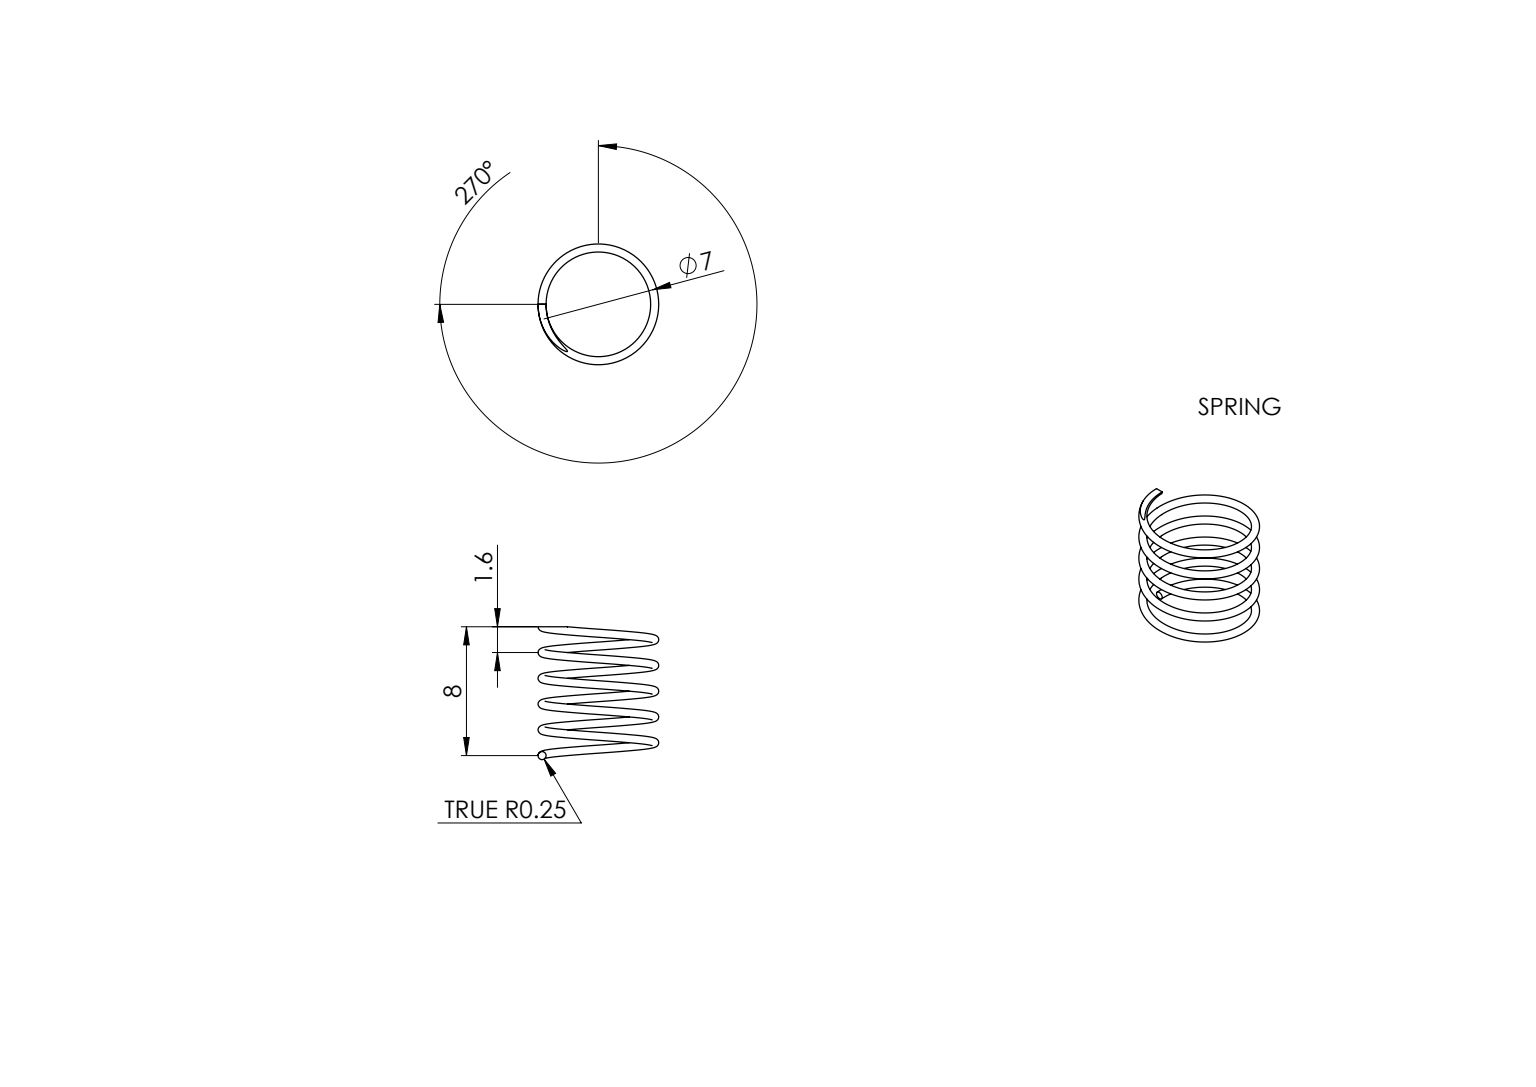
ISO-10303-21;
HEADER;
FILE_DESCRIPTION (('STEP AP214'),
    '1' );
FILE_NAME ('spring.step',
    '2026-10-27T10:49:47',
    ( '' ),
    ( '' ),
    'SwSTEP 2.0',
    'SolidWorks 2026',
    '' );
FILE_SCHEMA (( 'AUTOMOTIVE_DESIGN' ));
ENDSEC;

DATA;
#5=CARTESIAN_POINT ( 'NONE',  ( -2.108492589042352261, -1.550659073900639395, 2.134148098076933397 ) ) ;
#11=( NAMED_UNIT ( * ) SI_UNIT ( $, .STERADIAN. ) SOLID_ANGLE_UNIT ( ) );
#15=CARTESIAN_POINT ( 'NONE',  ( -2.593667801677444817, -2.017599804162952387E-16, 2.576081167903025104 ) ) ;
#18=CARTESIAN_POINT ( 'NONE',  ( -1.467888652719046449, -6.949340926099361049, 3.492485675378536047 ) ) ;
#25=CARTESIAN_POINT ( 'NONE',  ( 0.01814118441313990887, -6.550659073900639839, 3.500000000000000000 ) ) ;
#33=CARTESIAN_POINT ( 'NONE',  ( 3.492485675378536047, -0.9493409260993610488, 1.467888652719046672 ) ) ;
#36=CARTESIAN_POINT ( 'NONE',  ( 1.260781871532495657, -2.949340926099361937, -2.992485675378538268 ) ) ;
#40=CARTESIAN_POINT ( 'NONE',  ( 1.638713065079247855, -2.450659073900638862, -4.007514324621431534 ) ) ;
#50=CARTESIAN_POINT ( 'NONE',  ( 2.992485675378565357, -0.6506590739006395951, -1.260781871532430376 ) ) ;
#59=CARTESIAN_POINT ( 'NONE',  ( -2.110065146580993645, -1.191525181865938352E-11, 2.889420178070662093 ) ) ;
#61=CARTESIAN_POINT ( 'NONE',  ( -1.431606283892620235, -7.949340926099361049, -3.507514324621463953 ) ) ;
#62=CARTESIAN_POINT ( 'NONE',  ( -1.467888652719046449, -3.749340926099360871, 3.492485675378536047 ) ) ;
#69=CARTESIAN_POINT ( 'NONE',  ( 2.487701488670203354, -6.750659073900639129, 2.462045979635629323 ) ) ;
#77=CARTESIAN_POINT ( 'NONE',  ( -3.507514324621464397, -0.3493409260993610710, 1.431606283892619347 ) ) ;
#78=CARTESIAN_POINT ( 'NONE',  ( -3.000000000000000444, -5.049340926099361582, -0.01814118441320822922 ) ) ;
#82=CARTESIAN_POINT ( 'NONE',  ( 0.01814118441321938349, -1.449340926099360827, -4.000000000000000000 ) ) ;
#90=CARTESIAN_POINT ( 'NONE',  ( 2.134148098076933397, -5.150659073900639484, 2.108492589042352261 ) ) ;
#104=CARTESIAN_POINT ( 'NONE',  ( 3.492485675378536047, -7.349340926099362292, 1.467888652719046672 ) ) ;
#114=CARTESIAN_POINT ( 'NONE',  ( -4.000000000000000000, -7.750659073900639129, 0.01814118441313491634 ) ) ;
#122=CARTESIAN_POINT ( 'NONE',  ( -2.487701488670255312, -2.049340926099361582, 2.462045979635577808 ) ) ;
#125=CARTESIAN_POINT ( 'NONE',  ( 3.000000000000000444, -5.849340926099360516, 0.01814118441320859698 ) ) ;
#127=CARTESIAN_POINT ( 'NONE',  ( -1.674995433905599462, -0.5493409260993608045, 3.992485675378533383 ) ) ;
#138=CARTESIAN_POINT ( 'NONE',  ( 3.007514324621436863, -6.850659073900641438, 1.224499502706140719 ) ) ;
#139=ORIENTED_EDGE ( 'NONE', *, *, #8501, .F. ) ;
#149=CARTESIAN_POINT ( 'NONE',  ( 1.431606283892619125, -5.549340926099361582, 3.507514324621464397 ) ) ;
#152=CARTESIAN_POINT ( 'NONE',  ( -1.467888652719046449, -6.949340926099361049, 3.492485675378536047 ) ) ;
#155=CARTESIAN_POINT ( 'NONE',  ( 2.487701488670203354, -6.750659073900639129, 2.462045979635629323 ) ) ;
#156=AXIS2_PLACEMENT_3D ( 'NONE', #2203, #2343, #5173 ) ;
#161=CARTESIAN_POINT ( 'NONE',  ( -1.674995433905516196, -5.850659073900638774, -3.992485675378566690 ) ) ;
#169=CARTESIAN_POINT ( 'NONE',  ( 2.462045979635577364, -2.449340926099361049, 2.487701488670255312 ) ) ;
#171=CARTESIAN_POINT ( 'NONE',  ( 1.224499502706142273, -2.450659073900639751, -3.007514324621435531 ) ) ;
#174=CARTESIAN_POINT ( 'NONE',  ( -2.815599370228846876, -1.649340926099360560, -2.841254879263533262 ) ) ;
#177=CARTESIAN_POINT ( 'NONE',  ( 2.462045979635577364, -0.8493409260993610710, 2.487701488670255312 ) ) ;
#181=CARTESIAN_POINT ( 'NONE',  ( -1.674995433905599462, -5.349340926099361404, 3.992485675378533383 ) ) ;
#183=VERTEX_POINT ( 'NONE', #6311 ) ;
#185=CARTESIAN_POINT ( 'NONE',  ( 2.992485675378565357, -5.450659073900638418, -1.260781871532430376 ) ) ;
#195=CARTESIAN_POINT ( 'NONE',  ( 1.467888652719048226, -1.349340926099361182, -3.492485675378536047 ) ) ;
#203=CARTESIAN_POINT ( 'NONE',  ( 3.507514324621434199, -6.850659073900639662, 1.431606283892693066 ) ) ;
#211=CARTESIAN_POINT ( 'NONE',  ( -3.992485675378568022, -3.050659073900638951, 1.674995433905515529 ) ) ;
#219=CARTESIAN_POINT ( 'NONE',  ( -3.000000000000000444, 0.2493409260993606213, 0.01814118441314532468 ) ) ;
#223=CARTESIAN_POINT ( 'NONE',  ( 1.674995433905601239, -1.349340926099360960, -3.992485675378532939 ) ) ;
#224=( BOUNDED_SURFACE ( )  B_SPLINE_SURFACE ( 3, 2, ( 
 ( #862, #77, #7899, #2314, #3760, #7195, #3662, #33, #7151, #5702, #1518, #3711, #8682, #6487, #6589, #4994, #6536, #6398, #122, #8546, #2971, #5140, #169, #8636, #2266, #7944, #7851, #1565, #2618, #4787, #7676, #3958, #2660, #1914, #3403, #6785, #1117, #8281, #411, #1259, #1961, #1297, #6886, #559, #1872, #4052, #7630, #1212, #2704, #4098, #3259, #6231, #4005, #5387, #4739, #8237, #4140, #6931, #8418, #6085, #9063, #514, #3357, #3307, #3445, #7586, #5533, #6973, #6187, #6138, #8968, #5435, #5573, #8377, #463, #9015, #5482, #2004, #2569, #8330, #8920 ),
 ( #4830, #602, #6272, #4650, #9107, #2752, #7491, #4695, #1161, #7533, #6839, #4365, #5615, #2973, #6489, #3664, #5046, #6401, #684, #1520, #8590, #7198, #3576, #7811, #8508, #728, #7153, #36, #6809, #2176, #7901, #1345, #2887, #2133, #776, #4184, #7718, #5662, #7016, #7853, #8548, #822, #4269, #3622, #8463, #1428, #4996, #7105, #78, #1474, #642, #6445, #1385, #2796, #4956, #2091, #125, #4317, #5798, #3488, #2929, #5703, #5749, #3531, #2045, #2220, #4870, #6313, #9149, #6355, #2842, #4915, #7763, #4230, #7061, #6591, #5191, #5981, #6538, #4451, #7946 ),
 ( #219, #3207, #5284, #5143, #7290, #3762, #8823, #7381, #8131, #2459, #1568, #915, #8637, #3071, #6680, #1007, #355, #8084, #8778, #4505, #5890, #3856, #3021, #7433, #3902, #5845, #1059, #171, #864, #3808, #4549, #6723, #4409, #8684, #309, #2408, #3161, #1711, #7336, #2268, #2316, #8730, #5096, #7239, #4595, #2362, #8033, #1664, #962, #7985, #6634, #262, #3713, #1613, #1759, #3115, #5938, #5238, #3250, #4128, #3995, #6073, #6962, #4779, #402, #7666, #3299, #593, #4088, #3948, #6026, #2695, #2557, #4686, #1152, #3392, #7621, #5522, #6221, #5327, #1861 ),
 ( #1248, #8863, #5472, #6177, #1903, #7523, #6923, #8910, #4822, #1288, #5377, #2503, #6775, #7478, #1202, #1949, #8180, #1809, #8228, #549, #9004, #9051, #8319, #4731, #4640, #6828, #6126, #1108, #453, #1994, #8957, #2608, #5424, #8272, #7573, #4044, #6876, #504, #3347, #8368, #2650, #7093, #4259, #633, #1510, #1376, #3477, #4354, #2166, #7008, #5034, #675, #7189, #1460, #1332, #8539, #1419, #4219, #3565, #6434, #2744, #717, #3519, #4986, #5564, #9096, #7051, #8409, #25, #6389, #69, #5650, #7843, #6304, #2831, #2873, #9179, #4307, #5694, #2036, #7143 ),
 ( #4174, #766, #6345, #9141, #2785, #4859, #2920, #5737, #8498, #4903, #7891, #3608, #8582, #2210, #3436, #5605, #8450, #2077, #7754, #2120, #4946, #7707, #6265, #7802, #995, #5083, #6479, #6578, #8767, #952, #7371, #299, #2350, #211, #7279, #8718, #6624, #4494, #3153, #251, #5180, #1601, #4584, #5971, #3061, #8022, #2307, #5227, #906, #5881, #1654, #8675, #5785, #3102, #5129, #5835, #3842, #6668, #7325, #3801, #7937, #161, #1558, #7976, #5927, #8071, #3753, #8812, #7228, #2398, #811, #4442, #5275, #1701, #4538, #2449, #3011, #8119, #1748, #3654, #114 ),
 ( #2963, #8627, #2258, #4398, #855, #3702, #6527, #343, #1045, #3893, #6713, #3196, #7421, #4559, #1017, #7998, #366, #6735, #2514, #230, #1069, #8740, #877, #7444, #8143, #1625, #3171, #7346, #5154, #6601, #3727, #3911, #3215, #8045, #2374, #8873, #2468, #7394, #6688, #8094, #3079, #5901, #925, #3774, #3818, #5203, #6551, #6035, #1673, #5340, #2326, #181, #6643, #5993, #3865, #1722, #4516, #8189, #1818, #7251, #3035, #5292, #972, #272, #318, #5855, #4464, #8695, #7302, #3125, #5949, #2419, #8788, #5249, #8832, #1770, #4605, #1982, #8994, #8441, #625 ),
 ( #1940, #4813, #4769, #667, #3467, #4937, #6868, #6296, #6256, #3427, #9042, #9172, #1280, #5597, #3512, #7658, #2684, #5514, #4119, #2112, #7697, #6213, #8357, #6953, #7745, #8309, #583, #492, #9088, #7613, #3339, #2729, #1190, #7043, #6915, #5556, #8400, #1369, #9132, #6335, #4209, #6168, #2028, #4034, #4851, #2066, #2776, #2642, #4894, #1322, #4165, #6999, #2820, #1237, #5640, #8490, #4079, #5463, #539, #3380, #2954, #3690, #3052, #707, #4978, #6515, #1548, #152, #7218, #3645, #7795, #2158, #7879, #5869, #8709, #3745, #5727, #61, #5022, #2910, #8530 ) ),
 .UNSPECIFIED., .T., .F., .T. ) 
 B_SPLINE_SURFACE_WITH_KNOTS ( ( 4, 3, 4 ),
 ( 3, 2, 2, 2, 2, 2, 2, 2, 2, 2, 2, 2, 2, 2, 2, 2, 2, 2, 2, 2, 2, 2, 2, 2, 2, 2, 2, 2, 2, 2, 2, 2, 2, 2, 2, 2, 2, 2, 2, 2, 3 ),
 ( 0.000000000000000000, 0.5000000000000000000, 1.000000000000000000 ),
 ( 0.000000000000000000, 0.02500000000000000139, 0.05000000000000000278, 0.07499999999999999722, 0.1000000000000000056, 0.1250000000000000000, 0.1499999999999999944, 0.1749999999999999889, 0.2000000000000000111, 0.2250000000000000056, 0.2500000000000000000, 0.2750000000000000222, 0.2999999999999999889, 0.3250000000000000111, 0.3499999999999999778, 0.3750000000000000000, 0.4000000000000000222, 0.4249999999999999889, 0.4500000000000000111, 0.4749999999999999778, 0.5000000000000000000, 0.5250000000000000222, 0.5500000000000000444, 0.5749999999999999556, 0.5999999999999999778, 0.6250000000000000000, 0.6500000000000000222, 0.6750000000000000444, 0.6999999999999999556, 0.7249999999999999778, 0.7500000000000000000, 0.7750000000000000222, 0.8000000000000000444, 0.8249999999999999556, 0.8499999999999999778, 0.8750000000000000000, 0.9000000000000000222, 0.9250000000000000444, 0.9499999999999999556, 0.9749999999999999778, 1.000000000000000000 ),
 .UNSPECIFIED. ) 
 GEOMETRIC_REPRESENTATION_ITEM ( )  RATIONAL_B_SPLINE_SURFACE ( (
 ( 1.000000000000000000, 0.9238795325112867385, 1.000000000000000000, 0.9238795325112867385, 1.000000000000000000, 0.9238795325112867385, 1.000000000000000000, 0.9238795325112867385, 1.000000000000000000, 0.9238795325112867385, 1.000000000000000000, 0.9238795325112867385, 1.000000000000000000, 0.9238795325112867385, 1.000000000000000000, 0.9238795325112867385, 1.000000000000000000, 0.9238795325112867385, 1.000000000000000000, 0.9238795325112867385, 1.000000000000000000, 0.9238795325112867385, 1.000000000000000000, 0.9238795325112867385, 1.000000000000000000, 0.9238795325112867385, 1.000000000000000000, 0.9238795325112867385, 1.000000000000000000, 0.9238795325112867385, 1.000000000000000000, 0.9238795325112867385, 1.000000000000000000, 0.9238795325112867385, 1.000000000000000000, 0.9238795325112867385, 1.000000000000000000, 0.9238795325112867385, 1.000000000000000000, 0.9238795325112867385, 1.000000000000000000, 0.9238795325112867385, 1.000000000000000000, 0.9238795325112867385, 1.000000000000000000, 0.9238795325112867385, 1.000000000000000000, 0.9238795325112867385, 1.000000000000000000, 0.9238795325112867385, 1.000000000000000000, 0.9238795325112867385, 1.000000000000000000, 0.9238795325112867385, 1.000000000000000000, 0.9238795325112867385, 1.000000000000000000, 0.9238795325112867385, 1.000000000000000000, 0.9238795325112867385, 1.000000000000000000, 0.9238795325112867385, 1.000000000000000000, 0.9238795325112867385, 1.000000000000000000, 0.9238795325112867385, 1.000000000000000000, 0.9238795325112867385, 1.000000000000000000, 0.9238795325112867385, 1.000000000000000000, 0.9238795325112867385, 1.000000000000000000, 0.9238795325112867385, 1.000000000000000000, 0.9238795325112867385, 1.000000000000000000, 0.9238795325112867385, 1.000000000000000000, 0.9238795325112867385, 1.000000000000000000),
 ( 0.3333333333333333703, 0.3079598441704289313, 0.3333333333333333703, 0.3079598441704289313, 0.3333333333333333703, 0.3079598441704289313, 0.3333333333333333703, 0.3079598441704289313, 0.3333333333333333703, 0.3079598441704289313, 0.3333333333333333703, 0.3079598441704289313, 0.3333333333333333703, 0.3079598441704289313, 0.3333333333333333703, 0.3079598441704289313, 0.3333333333333333703, 0.3079598441704289313, 0.3333333333333333703, 0.3079598441704289313, 0.3333333333333333703, 0.3079598441704289313, 0.3333333333333333703, 0.3079598441704289313, 0.3333333333333333703, 0.3079598441704289313, 0.3333333333333333703, 0.3079598441704289313, 0.3333333333333333703, 0.3079598441704289313, 0.3333333333333333703, 0.3079598441704289313, 0.3333333333333333703, 0.3079598441704289313, 0.3333333333333333703, 0.3079598441704289313, 0.3333333333333333703, 0.3079598441704289313, 0.3333333333333333703, 0.3079598441704289313, 0.3333333333333333703, 0.3079598441704289313, 0.3333333333333333703, 0.3079598441704289313, 0.3333333333333333703, 0.3079598441704289313, 0.3333333333333333703, 0.3079598441704289313, 0.3333333333333333703, 0.3079598441704289313, 0.3333333333333333703, 0.3079598441704289313, 0.3333333333333333703, 0.3079598441704289313, 0.3333333333333333703, 0.3079598441704289313, 0.3333333333333333703, 0.3079598441704289313, 0.3333333333333333703, 0.3079598441704289313, 0.3333333333333333703, 0.3079598441704289313, 0.3333333333333333703, 0.3079598441704289313, 0.3333333333333333703, 0.3079598441704289313, 0.3333333333333333703, 0.3079598441704289313, 0.3333333333333333703, 0.3079598441704289313, 0.3333333333333333703, 0.3079598441704289313, 0.3333333333333333703, 0.3079598441704289313, 0.3333333333333333703, 0.3079598441704289313, 0.3333333333333333703, 0.3079598441704289313, 0.3333333333333333703, 0.3079598441704289313, 0.3333333333333333703),
 ( 0.3333333333333333703, 0.3079598441704289313, 0.3333333333333333703, 0.3079598441704289313, 0.3333333333333333703, 0.3079598441704289313, 0.3333333333333333703, 0.3079598441704289313, 0.3333333333333333703, 0.3079598441704289313, 0.3333333333333333703, 0.3079598441704289313, 0.3333333333333333703, 0.3079598441704289313, 0.3333333333333333703, 0.3079598441704289313, 0.3333333333333333703, 0.3079598441704289313, 0.3333333333333333703, 0.3079598441704289313, 0.3333333333333333703, 0.3079598441704289313, 0.3333333333333333703, 0.3079598441704289313, 0.3333333333333333703, 0.3079598441704289313, 0.3333333333333333703, 0.3079598441704289313, 0.3333333333333333703, 0.3079598441704289313, 0.3333333333333333703, 0.3079598441704289313, 0.3333333333333333703, 0.3079598441704289313, 0.3333333333333333703, 0.3079598441704289313, 0.3333333333333333703, 0.3079598441704289313, 0.3333333333333333703, 0.3079598441704289313, 0.3333333333333333703, 0.3079598441704289313, 0.3333333333333333703, 0.3079598441704289313, 0.3333333333333333703, 0.3079598441704289313, 0.3333333333333333703, 0.3079598441704289313, 0.3333333333333333703, 0.3079598441704289313, 0.3333333333333333703, 0.3079598441704289313, 0.3333333333333333703, 0.3079598441704289313, 0.3333333333333333703, 0.3079598441704289313, 0.3333333333333333703, 0.3079598441704289313, 0.3333333333333333703, 0.3079598441704289313, 0.3333333333333333703, 0.3079598441704289313, 0.3333333333333333703, 0.3079598441704289313, 0.3333333333333333703, 0.3079598441704289313, 0.3333333333333333703, 0.3079598441704289313, 0.3333333333333333703, 0.3079598441704289313, 0.3333333333333333703, 0.3079598441704289313, 0.3333333333333333703, 0.3079598441704289313, 0.3333333333333333703, 0.3079598441704289313, 0.3333333333333333703, 0.3079598441704289313, 0.3333333333333333703, 0.3079598441704289313, 0.3333333333333333703),
 ( 1.000000000000000000, 0.9238795325112867385, 1.000000000000000000, 0.9238795325112867385, 1.000000000000000000, 0.9238795325112867385, 1.000000000000000000, 0.9238795325112867385, 1.000000000000000000, 0.9238795325112867385, 1.000000000000000000, 0.9238795325112867385, 1.000000000000000000, 0.9238795325112867385, 1.000000000000000000, 0.9238795325112867385, 1.000000000000000000, 0.9238795325112867385, 1.000000000000000000, 0.9238795325112867385, 1.000000000000000000, 0.9238795325112867385, 1.000000000000000000, 0.9238795325112867385, 1.000000000000000000, 0.9238795325112867385, 1.000000000000000000, 0.9238795325112867385, 1.000000000000000000, 0.9238795325112867385, 1.000000000000000000, 0.9238795325112867385, 1.000000000000000000, 0.9238795325112867385, 1.000000000000000000, 0.9238795325112867385, 1.000000000000000000, 0.9238795325112867385, 1.000000000000000000, 0.9238795325112867385, 1.000000000000000000, 0.9238795325112867385, 1.000000000000000000, 0.9238795325112867385, 1.000000000000000000, 0.9238795325112867385, 1.000000000000000000, 0.9238795325112867385, 1.000000000000000000, 0.9238795325112867385, 1.000000000000000000, 0.9238795325112867385, 1.000000000000000000, 0.9238795325112867385, 1.000000000000000000, 0.9238795325112867385, 1.000000000000000000, 0.9238795325112867385, 1.000000000000000000, 0.9238795325112867385, 1.000000000000000000, 0.9238795325112867385, 1.000000000000000000, 0.9238795325112867385, 1.000000000000000000, 0.9238795325112867385, 1.000000000000000000, 0.9238795325112867385, 1.000000000000000000, 0.9238795325112867385, 1.000000000000000000, 0.9238795325112867385, 1.000000000000000000, 0.9238795325112867385, 1.000000000000000000, 0.9238795325112867385, 1.000000000000000000, 0.9238795325112867385, 1.000000000000000000, 0.9238795325112867385, 1.000000000000000000),
 ( 0.3333333333333333703, 0.3079598441704289313, 0.3333333333333333703, 0.3079598441704289313, 0.3333333333333333703, 0.3079598441704289313, 0.3333333333333333703, 0.3079598441704289313, 0.3333333333333333703, 0.3079598441704289313, 0.3333333333333333703, 0.3079598441704289313, 0.3333333333333333703, 0.3079598441704289313, 0.3333333333333333703, 0.3079598441704289313, 0.3333333333333333703, 0.3079598441704289313, 0.3333333333333333703, 0.3079598441704289313, 0.3333333333333333703, 0.3079598441704289313, 0.3333333333333333703, 0.3079598441704289313, 0.3333333333333333703, 0.3079598441704289313, 0.3333333333333333703, 0.3079598441704289313, 0.3333333333333333703, 0.3079598441704289313, 0.3333333333333333703, 0.3079598441704289313, 0.3333333333333333703, 0.3079598441704289313, 0.3333333333333333703, 0.3079598441704289313, 0.3333333333333333703, 0.3079598441704289313, 0.3333333333333333703, 0.3079598441704289313, 0.3333333333333333703, 0.3079598441704289313, 0.3333333333333333703, 0.3079598441704289313, 0.3333333333333333703, 0.3079598441704289313, 0.3333333333333333703, 0.3079598441704289313, 0.3333333333333333703, 0.3079598441704289313, 0.3333333333333333703, 0.3079598441704289313, 0.3333333333333333703, 0.3079598441704289313, 0.3333333333333333703, 0.3079598441704289313, 0.3333333333333333703, 0.3079598441704289313, 0.3333333333333333703, 0.3079598441704289313, 0.3333333333333333703, 0.3079598441704289313, 0.3333333333333333703, 0.3079598441704289313, 0.3333333333333333703, 0.3079598441704289313, 0.3333333333333333703, 0.3079598441704289313, 0.3333333333333333703, 0.3079598441704289313, 0.3333333333333333703, 0.3079598441704289313, 0.3333333333333333703, 0.3079598441704289313, 0.3333333333333333703, 0.3079598441704289313, 0.3333333333333333703, 0.3079598441704289313, 0.3333333333333333703, 0.3079598441704289313, 0.3333333333333333703),
 ( 0.3333333333333333703, 0.3079598441704289313, 0.3333333333333333703, 0.3079598441704289313, 0.3333333333333333703, 0.3079598441704289313, 0.3333333333333333703, 0.3079598441704289313, 0.3333333333333333703, 0.3079598441704289313, 0.3333333333333333703, 0.3079598441704289313, 0.3333333333333333703, 0.3079598441704289313, 0.3333333333333333703, 0.3079598441704289313, 0.3333333333333333703, 0.3079598441704289313, 0.3333333333333333703, 0.3079598441704289313, 0.3333333333333333703, 0.3079598441704289313, 0.3333333333333333703, 0.3079598441704289313, 0.3333333333333333703, 0.3079598441704289313, 0.3333333333333333703, 0.3079598441704289313, 0.3333333333333333703, 0.3079598441704289313, 0.3333333333333333703, 0.3079598441704289313, 0.3333333333333333703, 0.3079598441704289313, 0.3333333333333333703, 0.3079598441704289313, 0.3333333333333333703, 0.3079598441704289313, 0.3333333333333333703, 0.3079598441704289313, 0.3333333333333333703, 0.3079598441704289313, 0.3333333333333333703, 0.3079598441704289313, 0.3333333333333333703, 0.3079598441704289313, 0.3333333333333333703, 0.3079598441704289313, 0.3333333333333333703, 0.3079598441704289313, 0.3333333333333333703, 0.3079598441704289313, 0.3333333333333333703, 0.3079598441704289313, 0.3333333333333333703, 0.3079598441704289313, 0.3333333333333333703, 0.3079598441704289313, 0.3333333333333333703, 0.3079598441704289313, 0.3333333333333333703, 0.3079598441704289313, 0.3333333333333333703, 0.3079598441704289313, 0.3333333333333333703, 0.3079598441704289313, 0.3333333333333333703, 0.3079598441704289313, 0.3333333333333333703, 0.3079598441704289313, 0.3333333333333333703, 0.3079598441704289313, 0.3333333333333333703, 0.3079598441704289313, 0.3333333333333333703, 0.3079598441704289313, 0.3333333333333333703, 0.3079598441704289313, 0.3333333333333333703, 0.3079598441704289313, 0.3333333333333333703),
 ( 1.000000000000000000, 0.9238795325112867385, 1.000000000000000000, 0.9238795325112867385, 1.000000000000000000, 0.9238795325112867385, 1.000000000000000000, 0.9238795325112867385, 1.000000000000000000, 0.9238795325112867385, 1.000000000000000000, 0.9238795325112867385, 1.000000000000000000, 0.9238795325112867385, 1.000000000000000000, 0.9238795325112867385, 1.000000000000000000, 0.9238795325112867385, 1.000000000000000000, 0.9238795325112867385, 1.000000000000000000, 0.9238795325112867385, 1.000000000000000000, 0.9238795325112867385, 1.000000000000000000, 0.9238795325112867385, 1.000000000000000000, 0.9238795325112867385, 1.000000000000000000, 0.9238795325112867385, 1.000000000000000000, 0.9238795325112867385, 1.000000000000000000, 0.9238795325112867385, 1.000000000000000000, 0.9238795325112867385, 1.000000000000000000, 0.9238795325112867385, 1.000000000000000000, 0.9238795325112867385, 1.000000000000000000, 0.9238795325112867385, 1.000000000000000000, 0.9238795325112867385, 1.000000000000000000, 0.9238795325112867385, 1.000000000000000000, 0.9238795325112867385, 1.000000000000000000, 0.9238795325112867385, 1.000000000000000000, 0.9238795325112867385, 1.000000000000000000, 0.9238795325112867385, 1.000000000000000000, 0.9238795325112867385, 1.000000000000000000, 0.9238795325112867385, 1.000000000000000000, 0.9238795325112867385, 1.000000000000000000, 0.9238795325112867385, 1.000000000000000000, 0.9238795325112867385, 1.000000000000000000, 0.9238795325112867385, 1.000000000000000000, 0.9238795325112867385, 1.000000000000000000, 0.9238795325112867385, 1.000000000000000000, 0.9238795325112867385, 1.000000000000000000, 0.9238795325112867385, 1.000000000000000000, 0.9238795325112867385, 1.000000000000000000, 0.9238795325112867385, 1.000000000000000000, 0.9238795325112867385, 1.000000000000000000) ) ) 
 REPRESENTATION_ITEM ( '' )  SURFACE ( )  );
#227=CARTESIAN_POINT ( 'NONE',  ( -0.01814118441321365544, -0.6493409260993610044, 3.500000000000000000 ) ) ;
#230=CARTESIAN_POINT ( 'NONE',  ( -1.674995433905599462, -2.149340926099360782, 3.992485675378533383 ) ) ;
#234=CARTESIAN_POINT ( 'NONE',  ( -1.260781871532431708, -5.850659073900641438, -2.992485675378564469 ) ) ;
#240=CARTESIAN_POINT ( 'NONE',  ( -1.467888652719046449, -3.749340926099360871, 3.492485675378536047 ) ) ;
#251=CARTESIAN_POINT ( 'NONE',  ( 4.007514324621432422, -3.650659073900639040, 1.638713065079246078 ) ) ;
#254=ORIENTED_EDGE ( 'NONE', *, *, #8365, .F. ) ;
#262=CARTESIAN_POINT ( 'NONE',  ( -1.224499502706140497, -4.850659073900639662, 3.007514324621436863 ) ) ;
#266=DIRECTION ( 'NONE',  ( 0.000000000000000000, -0.9973637043974449279, -0.07256473765270717025 ) ) ;
#267=CARTESIAN_POINT ( 'NONE',  ( 0.01814118441321408565, -1.449340926099361271, -3.500000000000000000 ) ) ;
#272=CARTESIAN_POINT ( 'NONE',  ( -3.992485675378532939, -6.549340926099361582, -1.674995433905601683 ) ) ;
#276=CARTESIAN_POINT ( 'NONE',  ( 0.01814118441314514080, -4.950659073900641083, 3.000000000000000444 ) ) ;
#280=CARTESIAN_POINT ( 'NONE',  ( -1.041183273768722772, -0.07758948893217661180, 3.505490685814065088 ) ) ;
#285=CARTESIAN_POINT ( 'NONE',  ( -2.487701488670255312, -2.049340926099361582, 2.462045979635577808 ) ) ;
#295=AXIS2_PLACEMENT_3D ( 'NONE', #3494, #5755, #4370 ) ;
#299=CARTESIAN_POINT ( 'NONE',  ( -4.007514324621431534, -2.850659073900638774, -1.638713065079248521 ) ) ;
#309=CARTESIAN_POINT ( 'NONE',  ( -2.108492589042352261, -3.150659073900639484, 2.134148098076933397 ) ) ;
#318=CARTESIAN_POINT ( 'NONE',  ( -4.000000000000000000, -6.649340926099362115, -0.01814118441321865144 ) ) ;
#322=CARTESIAN_POINT ( 'NONE',  ( 0.01814118441313990887, -6.550659073900639839, 3.500000000000000000 ) ) ;
#329=EDGE_LOOP ( 'NONE', ( #5209, #4297, #1353, #1594, #6573 ) ) ;
#332=CARTESIAN_POINT ( 'NONE',  ( -0.01814118441321365544, -5.449340926099361937, 3.500000000000000000 ) ) ;
#341=DIRECTION ( 'NONE',  ( 0.000000000000000000, -0.000000000000000000, 1.000000000000000000 ) ) ;
#343=CARTESIAN_POINT ( 'NONE',  ( 3.992485675378533383, -0.9493409260993608267, 1.674995433905599462 ) ) ;
#355=CARTESIAN_POINT ( 'NONE',  ( -3.000000000000000444, -1.350659073900639440, 0.01814118441314532468 ) ) ;
#361=CARTESIAN_POINT ( 'NONE',  ( -3.500000000000000000, -0.2493409260993610654, -0.01814118441321343686 ) ) ;
#364=PRODUCT_CONTEXT ( 'NONE', #1831, 'mechanical' ) ;
#366=CARTESIAN_POINT ( 'NONE',  ( -4.000000000000000000, -1.849340926099360738, -0.01814118441321865144 ) ) ;
#371=CARTESIAN_POINT ( 'NONE',  ( 1.431606283892694842, -5.650659073900638596, -3.507514324621434199 ) ) ;
#380=CARTESIAN_POINT ( 'NONE',  ( 0.01814118441321408565, -7.849340926099360516, -3.500000000000000000 ) ) ;
#395=CARTESIAN_POINT ( 'NONE',  ( -2.841254879263533262, -0.4493409260993607157, 2.815599370228847764 ) ) ;
#402=CARTESIAN_POINT ( 'NONE',  ( -3.000000000000000444, -6.150659073900639484, 0.01814118441314532468 ) ) ;
#411=CARTESIAN_POINT ( 'NONE',  ( 2.462045979635577364, -4.049340926099360694, 2.487701488670255312 ) ) ;
#414=CARTESIAN_POINT ( 'NONE',  ( 3.492485675378566690, -7.050659073900641616, -1.467888652718972287 ) ) ;
#420=CARTESIAN_POINT ( 'NONE',  ( 3.492485675378566690, -0.6506590739006392621, -1.467888652718972287 ) ) ;
#426=CARTESIAN_POINT ( 'NONE',  ( -1.260781871532494103, -0.5493409260993613596, 2.992485675378538712 ) ) ;
#444=CARTESIAN_POINT ( 'NONE',  ( -1.638713065079163034, -6.349340926099361404, -4.007514324621466173 ) ) ;
#453=CARTESIAN_POINT ( 'NONE',  ( -0.01814118441313947866, -2.550659073900638951, -3.500000000000000000 ) ) ;
#463=CARTESIAN_POINT ( 'NONE',  ( 2.487701488670255756, -7.649340926099361226, -2.462045979635577364 ) ) ;
#466=CARTESIAN_POINT ( 'NONE',  ( 2.462045979635629767, -3.950659073900639751, -2.487701488670203354 ) ) ;
#470=CARTESIAN_POINT ( 'NONE',  ( 2.487701488670203354, -3.550659073900638951, 2.462045979635629323 ) ) ;
#477=CARTESIAN_POINT ( 'NONE',  ( -0.01814118441321365544, -7.049340926099361582, 3.500000000000000000 ) ) ;
#492=CARTESIAN_POINT ( 'NONE',  ( 1.467888652719048226, -2.949340926099361493, -3.492485675378536047 ) ) ;
#493=CARTESIAN_POINT ( 'NONE',  ( -2.815599370228846876, -6.449340926099361049, -2.841254879263533262 ) ) ;
#496=ADVANCED_FACE ( 'NONE', ( #7809 ), #224, .T. ) ;
#504=CARTESIAN_POINT ( 'NONE',  ( 1.467888652718972731, -3.450659073900638862, 3.492485675378566246 ) ) ;
#509=CARTESIAN_POINT ( 'NONE',  ( -3.507514324621464397, -6.749340926099361759, 1.431606283892619569 ) ) ;
#514=CARTESIAN_POINT ( 'NONE',  ( -1.431606283892620235, -6.349340926099360516, -3.507514324621463953 ) ) ;
#518=CARTESIAN_POINT ( 'NONE',  ( 2.487701488670203354, -3.550659073900638951, 2.462045979635629323 ) ) ;
#522=CARTESIAN_POINT ( 'NONE',  ( 3.500000000000000000, -5.350659073900638774, -0.01814118441313969030 ) ) ;
#527=CARTESIAN_POINT ( 'NONE',  ( 2.462045979635577364, -7.249340926099360871, 2.487701488670255312 ) ) ;
#531=( BOUNDED_CURVE ( )  B_SPLINE_CURVE ( 2, ( #361, #7438, #3211, #2413, #227, #6638, #177, #5198, #7991, #1813, #7388, #1621, #267, #6730, #5244, #8784, #8088, #2368, #5288, #7341, #5942, #966, #4644, #871, #4458, #3860, #6682, #4600, #1715, #3075, #4512, #8690, #3029, #7296, #6029, #920, #4554, #3166, #3770, #3720, #8040, #5896, #6545, #3120, #1765, #8828, #8736, #3813, #5987, #2463, #8137, #8868, #6597, #1063, #3907, #5851, #2507, #1669, #5569, #2748, #554, #3953, #4092, #4782, #1293, #509, #3397, #1999, #2700, #8276, #6078, #3352, #4134, #1113, #6182, #6131, #5528, #6225, #8414, #6928, #7624 ),
 .UNSPECIFIED., .F., .T. ) 
 B_SPLINE_CURVE_WITH_KNOTS ( ( 3, 2, 2, 2, 2, 2, 2, 2, 2, 2, 2, 2, 2, 2, 2, 2, 2, 2, 2, 2, 2, 2, 2, 2, 2, 2, 2, 2, 2, 2, 2, 2, 2, 2, 2, 2, 2, 2, 2, 2, 3 ),
 ( 0.000000000000000000, 0.02500000000000000139, 0.05000000000000000278, 0.07499999999999999722, 0.1000000000000000056, 0.1250000000000000000, 0.1499999999999999944, 0.1749999999999999889, 0.2000000000000000111, 0.2250000000000000056, 0.2500000000000000000, 0.2750000000000000222, 0.2999999999999999889, 0.3250000000000000111, 0.3499999999999999778, 0.3750000000000000000, 0.4000000000000000222, 0.4249999999999999889, 0.4500000000000000111, 0.4749999999999999778, 0.5000000000000000000, 0.5250000000000000222, 0.5500000000000000444, 0.5749999999999999556, 0.5999999999999999778, 0.6250000000000000000, 0.6500000000000000222, 0.6750000000000000444, 0.6999999999999999556, 0.7249999999999999778, 0.7500000000000000000, 0.7750000000000000222, 0.8000000000000000444, 0.8249999999999999556, 0.8499999999999999778, 0.8750000000000000000, 0.9000000000000000222, 0.9250000000000000444, 0.9499999999999999556, 0.9749999999999999778, 1.000000000000000000 ),
 .UNSPECIFIED. ) 
 CURVE ( )  GEOMETRIC_REPRESENTATION_ITEM ( )  RATIONAL_B_SPLINE_CURVE ( ( 1.000000000000000000, 0.9238795325112867385, 1.000000000000000000, 0.9238795325112867385, 1.000000000000000000, 0.9238795325112867385, 1.000000000000000000, 0.9238795325112867385, 1.000000000000000000, 0.9238795325112867385, 1.000000000000000000, 0.9238795325112867385, 1.000000000000000000, 0.9238795325112867385, 1.000000000000000000, 0.9238795325112867385, 1.000000000000000000, 0.9238795325112867385, 1.000000000000000000, 0.9238795325112867385, 1.000000000000000000, 0.9238795325112867385, 1.000000000000000000, 0.9238795325112867385, 1.000000000000000000, 0.9238795325112867385, 1.000000000000000000, 0.9238795325112867385, 1.000000000000000000, 0.9238795325112867385, 1.000000000000000000, 0.9238795325112867385, 1.000000000000000000, 0.9238795325112867385, 1.000000000000000000, 0.9238795325112867385, 1.000000000000000000, 0.9238795325112867385, 1.000000000000000000, 0.9238795325112867385, 1.000000000000000000, 0.9238795325112867385, 1.000000000000000000, 0.9238795325112867385, 1.000000000000000000, 0.9238795325112867385, 1.000000000000000000, 0.9238795325112867385, 1.000000000000000000, 0.9238795325112867385, 1.000000000000000000, 0.9238795325112867385, 1.000000000000000000, 0.9238795325112867385, 1.000000000000000000, 0.9238795325112867385, 1.000000000000000000, 0.9238795325112867385, 1.000000000000000000, 0.9238795325112867385, 1.000000000000000000, 0.9238795325112867385, 1.000000000000000000, 0.9238795325112867385, 1.000000000000000000, 0.9238795325112867385, 1.000000000000000000, 0.9238795325112867385, 1.000000000000000000, 0.9238795325112867385, 1.000000000000000000, 0.9238795325112867385, 1.000000000000000000, 0.9238795325112867385, 1.000000000000000000, 0.9238795325112867385, 1.000000000000000000, 0.9238795325112867385, 1.000000000000000000, 0.9238795325112867385, 1.000000000000000000 ) ) 
 REPRESENTATION_ITEM ( '' )  );
#539=CARTESIAN_POINT ( 'NONE',  ( 2.487701488670255756, -6.049340926099361582, -2.462045979635577364 ) ) ;
#540=CARTESIAN_POINT ( 'NONE',  ( 3.992485675378533383, -5.749340926099361759, 1.674995433905599462 ) ) ;
#542=ADVANCED_BREP_SHAPE_REPRESENTATION ( '', ( #8451, #888 ), #3388 ) ;
#549=CARTESIAN_POINT ( 'NONE',  ( -1.431606283892693066, -1.650659073900638818, 3.507514324621434199 ) ) ;
#554=CARTESIAN_POINT ( 'NONE',  ( 0.01814118441321408565, -6.249340926099360871, -3.500000000000000000 ) ) ;
#559=CARTESIAN_POINT ( 'NONE',  ( 1.467888652719048226, -4.549340926099360694, -3.492485675378536047 ) ) ;
#562=CARTESIAN_POINT ( 'NONE',  ( 2.815599370228907716, -2.350659073900638774, -2.841254879263473310 ) ) ;
#569=CARTESIAN_POINT ( 'NONE',  ( -0.01814118441320841310, -0.6493409260993614485, 3.000000000000000444 ) ) ;
#583=CARTESIAN_POINT ( 'NONE',  ( 2.487701488670255756, -2.849340926099361404, -2.462045979635577364 ) ) ;
#584=CARTESIAN_POINT ( 'NONE',  ( 3.500000000000000000, -2.649340926099361226, 0.01814118441321387054 ) ) ;
#593=CARTESIAN_POINT ( 'NONE',  ( -1.224499502706140497, -6.450659073900641971, 3.007514324621436863 ) ) ;
#602=CARTESIAN_POINT ( 'NONE',  ( -3.007514324621463508, -0.3493409260993614596, 1.224499502706077658 ) ) ;
#605=CARTESIAN_POINT ( 'NONE',  ( -2.815599370228907272, -4.750659073900638241, 2.841254879263473754 ) ) ;
#614=CARTESIAN_POINT ( 'NONE',  ( -1.224499502706077880, -6.349340926099361404, -3.007514324621463064 ) ) ;
#622=CARTESIAN_POINT ( 'NONE',  ( -2.487701488670255312, -0.4493409260993610488, 2.462045979635577808 ) ) ;
#625=CARTESIAN_POINT ( 'NONE',  ( -4.000000000000000000, -8.249340926099360871, -0.01814118441321865144 ) ) ;
#626=CARTESIAN_POINT ( 'NONE',  ( 3.500000000000000000, -1.049340926099360916, 0.01814118441321387054 ) ) ;
#633=CARTESIAN_POINT ( 'NONE',  ( 1.431606283892694842, -4.050659073900638951, -3.507514324621434199 ) ) ;
#642=CARTESIAN_POINT ( 'NONE',  ( -2.134148098076978251, -5.249340926099361759, 2.108492589042307408 ) ) ;
#646=CARTESIAN_POINT ( 'NONE',  ( -1.674995433905516196, -4.250659073900640017, -3.992485675378566690 ) ) ;
#650=CARTESIAN_POINT ( 'NONE',  ( -2.351851292788933456, -1.491716277578878685E-16, 2.391493231060961566 ) ) ;
#658=CARTESIAN_POINT ( 'NONE',  ( 2.108492589042307408, -7.249340926099360871, 2.134148098076978251 ) ) ;
#667=CARTESIAN_POINT ( 'NONE',  ( -1.467888652719046449, -0.5493409260993611376, 3.492485675378536047 ) ) ;
#668=CARTESIAN_POINT ( 'NONE',  ( 3.507514324621465285, -4.349340926099361404, -1.431606283892619125 ) ) ;
#675=CARTESIAN_POINT ( 'NONE',  ( -1.431606283892693066, -4.850659073900638774, 3.507514324621434199 ) ) ;
#684=CARTESIAN_POINT ( 'NONE',  ( -2.134148098076978251, -2.049340926099361138, 2.108492589042307408 ) ) ;
#688=CARTESIAN_POINT ( 'NONE',  ( -0.01814118441313417734, -2.550659073900638951, -4.000000000000000000 ) ) ;
#696=CARTESIAN_POINT ( 'NONE',  ( 0.01814118441320878086, -6.249340926099361759, -3.000000000000000444 ) ) ;
#705=CARTESIAN_POINT ( 'NONE',  ( -2.019217148918400095, -3.217773791669851107E-17, 2.923265991829747446 ) ) ;
#707=CARTESIAN_POINT ( 'NONE',  ( -3.492485675378536047, -6.549340926099363358, -1.467888652719048670 ) ) ;
#708=CARTESIAN_POINT ( 'NONE',  ( -0.01814118441321365544, -3.849340926099361404, 3.500000000000000000 ) ) ;
#717=CARTESIAN_POINT ( 'NONE',  ( -1.467888652718973619, -5.850659073900639662, -3.492485675378565801 ) ) ;
#728=CARTESIAN_POINT ( 'NONE',  ( 3.007514324621463508, -2.749340926099361759, -1.224499502706076770 ) ) ;
#731=CARTESIAN_POINT ( 'NONE',  ( 1.638713065079247855, -0.8506590739006385515, -4.007514324621431534 ) ) ;
#740=CARTESIAN_POINT ( 'NONE',  ( -1.260781871532431708, -1.050659073900639617, -2.992485675378564469 ) ) ;
#748=( NAMED_UNIT ( * ) PLANE_ANGLE_UNIT ( ) SI_UNIT ( $, .RADIAN. ) );
#755=CARTESIAN_POINT ( 'NONE',  ( 2.487701488670255756, -4.449340926099361937, -2.462045979635577364 ) ) ;
#758=CARTESIAN_POINT ( 'NONE',  ( -1.467888652718973841, -5.850659073900639662, -3.492485675378565801 ) ) ;
#766=CARTESIAN_POINT ( 'NONE',  ( -3.992485675378568022, 0.1493409260993615040, 1.674995433905515529 ) ) ;
#776=CARTESIAN_POINT ( 'NONE',  ( -2.134148098076978251, -3.649340926099361671, 2.108492589042307408 ) ) ;
#779=CARTESIAN_POINT ( 'NONE',  ( -2.841254879263473310, -7.550659073900639839, -2.815599370228907716 ) ) ;
#790=CARTESIAN_POINT ( 'NONE',  ( -1.260781871532431708, -4.250659073900640017, -2.992485675378564469 ) ) ;
#802=CARTESIAN_POINT ( 'NONE',  ( 2.487701488670255756, -7.649340926099361226, -2.462045979635577364 ) ) ;
#804=CARTESIAN_POINT ( 'NONE',  ( 1.431606283892694620, -5.650659073900638596, -3.507514324621433754 ) ) ;
#811=CARTESIAN_POINT ( 'NONE',  ( 2.841254879263473310, -6.750659073900638241, 2.815599370228907272 ) ) ;
#822=CARTESIAN_POINT ( 'NONE',  ( 3.007514324621463508, -4.349340926099361404, -1.224499502706076770 ) ) ;
#825=CARTESIAN_POINT ( 'NONE',  ( 0.01814118441321938349, -4.649340926099361226, -4.000000000000000000 ) ) ;
#834=CARTESIAN_POINT ( 'NONE',  ( 2.992485675378565357, -7.050659073900639839, -1.260781871532430376 ) ) ;
#840=CARTESIAN_POINT ( 'NONE',  ( 3.500000000000000000, -2.649340926099361226, 0.01814118441321387054 ) ) ;
#845=VERTEX_POINT ( 'NONE', #3118 ) ;
#855=CARTESIAN_POINT ( 'NONE',  ( -0.01814118441321889430, -0.6493409260993606713, 4.000000000000000000 ) ) ;
#862=CARTESIAN_POINT ( 'NONE',  ( -3.500000000000000000, -0.2493409260993610654, -0.01814118441321344033 ) ) ;
#864=CARTESIAN_POINT ( 'NONE',  ( -0.01814118441314477650, -2.550659073900638951, -3.000000000000000444 ) ) ;
#866=CARTESIAN_POINT ( 'NONE',  ( 2.815599370228907716, -7.150659073900638596, -2.841254879263473310 ) ) ;
#871=CARTESIAN_POINT ( 'NONE',  ( 3.492485675378535603, -2.549340926099361138, 1.467888652719046672 ) ) ;
#872=EDGE_CURVE ( 'NONE', #8537, #7146, #935, .T. ) ;
#877=CARTESIAN_POINT ( 'NONE',  ( 2.815599370228847320, -2.449340926099361049, 2.841254879263533262 ) ) ;
#880=( GEOMETRIC_REPRESENTATION_CONTEXT ( 3 ) GLOBAL_UNCERTAINTY_ASSIGNED_CONTEXT ( ( #5144 ) ) GLOBAL_UNIT_ASSIGNED_CONTEXT ( ( #5512, #7423, #9170 ) ) REPRESENTATION_CONTEXT ( 'NONE', 'WORKASPACE' ) );
#882=CARTESIAN_POINT ( 'NONE',  ( -2.134148098076932953, -7.550659073900640728, -2.108492589042352705 ) ) ;
#885=EDGE_CURVE ( 'NONE', #8537, #845, #3165, .T. ) ;
#888=AXIS2_PLACEMENT_3D ( 'NONE', #4026, #9081, #6861 ) ;
#892=CARTESIAN_POINT ( 'NONE',  ( -2.487701488670255312, -3.649340926099361226, 2.462045979635577808 ) ) ;
#897=CARTESIAN_POINT ( 'NONE',  ( 3.500000000000000000, -6.950659073900639306, -0.01814118441313969030 ) ) ;
#906=CARTESIAN_POINT ( 'NONE',  ( -4.000000000000000000, -4.550659073900638951, 0.01814118441313491634 ) ) ;
#915=CARTESIAN_POINT ( 'NONE',  ( 1.224499502706142273, -0.8506590739006396618, -3.007514324621435531 ) ) ;
#917=CARTESIAN_POINT ( 'NONE',  ( 4.007514324621432422, -6.850659073900641438, 1.638713065079246078 ) ) ;
#920=CARTESIAN_POINT ( 'NONE',  ( -1.467888652719046449, -3.749340926099361315, 3.492485675378535603 ) ) ;
#925=CARTESIAN_POINT ( 'NONE',  ( 2.841254879263533262, -4.449340926099361937, -2.815599370228847320 ) ) ;
#929=CARTESIAN_POINT ( 'NONE',  ( -2.134148098076932953, -5.950659073900640195, -2.108492589042352705 ) ) ;
#935=CIRCLE ( 'NONE', #5240, 0.2499999999999998335 ) ;
#940=CARTESIAN_POINT ( 'NONE',  ( -3.500000000000000000, -3.449340926099361049, -0.01814118441321344033 ) ) ;
#952=CARTESIAN_POINT ( 'NONE',  ( -1.674995433905516196, -2.650659073900639040, -3.992485675378566690 ) ) ;
#962=CARTESIAN_POINT ( 'NONE',  ( -3.000000000000000444, -4.550659073900638951, 0.01814118441314532468 ) ) ;
#966=CARTESIAN_POINT ( 'NONE',  ( 1.431606283892619347, -2.349340926099361404, 3.507514324621464397 ) ) ;
#972=CARTESIAN_POINT ( 'NONE',  ( -2.815599370228846876, -6.449340926099361049, -2.841254879263533262 ) ) ;
#976=CARTESIAN_POINT ( 'NONE',  ( 1.260781871532430598, -5.050659073900640728, 2.992485675378564469 ) ) ;
#979=CARTESIAN_POINT ( 'NONE',  ( -1.467888652718973841, -1.050659073900639173, -3.492485675378565801 ) ) ;
#983=CARTESIAN_POINT ( 'NONE',  ( -3.492485675378536047, -3.349340926099361404, -1.467888652719048670 ) ) ;
#995=CARTESIAN_POINT ( 'NONE',  ( 4.000000000000000000, -2.150659073900639040, -0.01814118441313441674 ) ) ;
#1007=CARTESIAN_POINT ( 'NONE',  ( -3.007514324621435531, -1.250659073900639573, -1.224499502706142273 ) ) ;
#1017=CARTESIAN_POINT ( 'NONE',  ( -2.815599370228846876, -1.649340926099360560, -2.841254879263533262 ) ) ;
#1021=CARTESIAN_POINT ( 'NONE',  ( 0.01814118441313990887, -4.950659073900639306, 3.500000000000000000 ) ) ;
#1025=CARTESIAN_POINT ( 'NONE',  ( 0.01814118441313990887, -0.1506590739006389568, 3.500000000000000000 ) ) ;
#1031=CARTESIAN_POINT ( 'NONE',  ( -3.500000000000000000, -5.049340926099361582, -0.01814118441321344033 ) ) ;
#1042=CLOSED_SHELL ( 'NONE', ( #5130, #1686, #496, #8751, #6627 ) ) ;
#1045=CARTESIAN_POINT ( 'NONE',  ( 4.000000000000000000, -1.049340926099360916, 0.01814118441321914063 ) ) ;
#1059=CARTESIAN_POINT ( 'NONE',  ( 2.108492589042352705, -2.350659073900639218, -2.134148098076933397 ) ) ;
#1063=CARTESIAN_POINT ( 'NONE',  ( 1.431606283892619347, -5.549340926099361582, 3.507514324621464397 ) ) ;
#1069=CARTESIAN_POINT ( 'NONE',  ( -0.01814118441321889430, -2.249340926099360427, 4.000000000000000000 ) ) ;
#1073=CARTESIAN_POINT ( 'NONE',  ( -2.462045979635629323, -4.750659073900639129, 2.487701488670203798 ) ) ;
#1084=CARTESIAN_POINT ( 'NONE',  ( -2.992485675378538268, -4.949340926099361937, -1.260781871532495879 ) ) ;
#1090=CARTESIAN_POINT ( 'NONE',  ( -2.075653704136731559, -4.858300672349190065E-16, 2.699248787648522274 ) ) ;
#1092=ORIENTED_EDGE ( 'NONE', *, *, #3526, .F. ) ;
#1094=DIRECTION ( 'NONE',  ( 0.000000000000000000, 1.000000000000000000, 0.000000000000000000 ) ) ;
#1100=CARTESIAN_POINT ( 'NONE',  ( -0.01814118441321889430, -3.849340926099360960, 4.000000000000000000 ) ) ;
#1108=CARTESIAN_POINT ( 'NONE',  ( 1.431606283892694842, -2.450659073900638862, -3.507514324621434199 ) ) ;
#1113=CARTESIAN_POINT ( 'NONE',  ( 3.507514324621465285, -7.549340926099361582, -1.431606283892619347 ) ) ;
#1117=CARTESIAN_POINT ( 'NONE',  ( -0.01814118441321365544, -3.849340926099361404, 3.500000000000000000 ) ) ;
#1121=CARTESIAN_POINT ( 'NONE',  ( -1.431606283892693066, -6.450659073900639306, 3.507514324621434199 ) ) ;
#1126=CARTESIAN_POINT ( 'NONE',  ( 2.462045979635629767, -3.950659073900639751, -2.487701488670203354 ) ) ;
#1132=CARTESIAN_POINT ( 'NONE',  ( 2.487701488670255756, -7.649340926099361226, -2.462045979635577364 ) ) ;
#1145=CARTESIAN_POINT ( 'NONE',  ( 0.01814118441321938349, -7.849340926099360516, -4.000000000000000000 ) ) ;
#1152=CARTESIAN_POINT ( 'NONE',  ( 2.108492589042352705, -7.150659073900638596, -2.134148098076933397 ) ) ;
#1161=CARTESIAN_POINT ( 'NONE',  ( 3.000000000000000444, -1.049340926099361582, 0.01814118441320859698 ) ) ;
#1164=CARTESIAN_POINT ( 'NONE',  ( -2.487701488670202910, -5.950659073900639306, -2.462045979635629767 ) ) ;
#1170=CARTESIAN_POINT ( 'NONE',  ( -2.487701488670202910, -1.150659073900638818, -2.462045979635629767 ) ) ;
#1176=CARTESIAN_POINT ( 'NONE',  ( 1.260781871532495657, -2.949340926099361937, -2.992485675378538268 ) ) ;
#1180=CARTESIAN_POINT ( 'NONE',  ( -2.261299776309945386, -1.321938709600328683E-17, 2.495489592912619070 ) ) ;
#1190=CARTESIAN_POINT ( 'NONE',  ( -3.500000000000000000, -3.449340926099361049, -0.01814118441321344033 ) ) ;
#1192=CARTESIAN_POINT ( 'NONE',  ( -2.462045979635576920, -1.649340926099361004, -2.487701488670255756 ) ) ;
#1202=CARTESIAN_POINT ( 'NONE',  ( -2.487701488670202910, -1.150659073900638818, -2.462045979635629767 ) ) ;
#1212=CARTESIAN_POINT ( 'NONE',  ( -3.492485675378536047, -4.949340926099361049, -1.467888652719048670 ) ) ;
#1215=CARTESIAN_POINT ( 'NONE',  ( 1.467888652718972731, -5.050659073900638063, 3.492485675378566246 ) ) ;
#1219=CARTESIAN_POINT ( 'NONE',  ( 0.01814118441313990887, -4.950659073900639306, 3.500000000000000000 ) ) ;
#1224=CARTESIAN_POINT ( 'NONE',  ( 2.992485675378538712, -4.149340926099362115, 1.260781871532494103 ) ) ;
#1237=CARTESIAN_POINT ( 'NONE',  ( 1.431606283892619125, -5.549340926099361582, 3.507514324621464397 ) ) ;
#1238=CARTESIAN_POINT ( 'NONE',  ( -1.431606283892620235, -1.549340926099361138, -3.507514324621463953 ) ) ;
#1248=CARTESIAN_POINT ( 'NONE',  ( -3.500000000000000000, 0.2493409260993610654, 0.01814118441314012051 ) ) ;
#1259=CARTESIAN_POINT ( 'NONE',  ( 3.492485675378536047, -4.149340926099361226, 1.467888652719046672 ) ) ;
#1262=CARTESIAN_POINT ( 'NONE',  ( 4.000000000000000000, -5.350659073900637885, -0.01814118441313441674 ) ) ;
#1270=CARTESIAN_POINT ( 'NONE',  ( 3.500000000000000000, -7.449340926099361937, 0.01814118441321387054 ) ) ;
#1280=CARTESIAN_POINT ( 'NONE',  ( 0.01814118441321408565, -1.449340926099361271, -3.500000000000000000 ) ) ;
#1281=CARTESIAN_POINT ( 'NONE',  ( 1.431606283892619125, -2.349340926099361848, 3.507514324621464397 ) ) ;
#1288=CARTESIAN_POINT ( 'NONE',  ( 3.492485675378566690, -0.6506590739006391511, -1.467888652718972287 ) ) ;
#1293=CARTESIAN_POINT ( 'NONE',  ( -3.500000000000000000, -6.649340926099361226, -0.01814118441321344033 ) ) ;
#1297=CARTESIAN_POINT ( 'NONE',  ( 3.507514324621465285, -4.349340926099361404, -1.431606283892619125 ) ) ;
#1301=CARTESIAN_POINT ( 'NONE',  ( -2.841254879263473310, -1.150659073900638374, -2.815599370228907716 ) ) ;
#1309=CARTESIAN_POINT ( 'NONE',  ( -1.224499502706140497, -1.650659073900639484, 3.007514324621436863 ) ) ;
#1319=CARTESIAN_POINT ( 'NONE',  ( -3.500000000000000000, -0.2493409260993610654, -0.01814118441321344033 ) ) ;
#1322=CARTESIAN_POINT ( 'NONE',  ( -3.507514324621464397, -5.149340926099360338, 1.431606283892619347 ) ) ;
#1323=CARTESIAN_POINT ( 'NONE',  ( -2.487701488670255312, -0.4493409260993610488, 2.462045979635577808 ) ) ;
#1332=CARTESIAN_POINT ( 'NONE',  ( 2.487701488670203354, -5.150659073900639484, 2.462045979635629323 ) ) ;
#1345=CARTESIAN_POINT ( 'NONE',  ( -2.992485675378538268, -3.349340926099362292, -1.260781871532495879 ) ) ;
#1349=CARTESIAN_POINT ( 'NONE',  ( -1.638713065079245634, -3.250659073900639129, 4.007514324621432422 ) ) ;
#1353=ORIENTED_EDGE ( 'NONE', *, *, #3526, .T. ) ;
#1357=CARTESIAN_POINT ( 'NONE',  ( -2.992485675378538268, -6.549340926099361582, -1.260781871532495879 ) ) ;
#1369=CARTESIAN_POINT ( 'NONE',  ( 1.431606283892619125, -3.949340926099361049, 3.507514324621464397 ) ) ;
#1370=CARTESIAN_POINT ( 'NONE',  ( -0.01814118441321365544, -7.049340926099361582, 3.500000000000000000 ) ) ;
#1376=CARTESIAN_POINT ( 'NONE',  ( -1.467888652718973619, -4.250659073900639129, -3.492485675378565801 ) ) ;
#1385=CARTESIAN_POINT ( 'NONE',  ( -0.01814118441320841310, -5.449340926099361937, 3.000000000000000444 ) ) ;
#1390=CARTESIAN_POINT ( 'NONE',  ( 0.01814118441313467001, -0.1506590739006384849, 4.000000000000000000 ) ) ;
#1400=CARTESIAN_POINT ( 'NONE',  ( 0.01814118441320878086, -7.849340926099363180, -3.000000000000000444 ) ) ;
#1410=CARTESIAN_POINT ( 'NONE',  ( -1.931223450958591048, -1.125130374610754074E-16, 2.930832316995867437 ) ) ;
#1419=CARTESIAN_POINT ( 'NONE',  ( 3.500000000000000000, -5.350659073900638774, -0.01814118441313969030 ) ) ;
#1428=CARTESIAN_POINT ( 'NONE',  ( -1.224499502706077880, -4.749340926099361759, -3.007514324621463064 ) ) ;
#1431=CARTESIAN_POINT ( 'NONE',  ( -0.01814118441313417734, -0.9506590739006385293, -4.000000000000000000 ) ) ;
#1438=CARTESIAN_POINT ( 'NONE',  ( -2.108492589042306964, -8.049340926099361582, -2.134148098076978251 ) ) ;
#1449=CARTESIAN_POINT ( 'NONE',  ( -3.709488398121285169, -3.053917841153453545E-13, 0.6142436145054751551 ) ) ;
#1454=CARTESIAN_POINT ( 'NONE',  ( 2.462045979635629767, -7.150659073900639484, -2.487701488670203354 ) ) ;
#1460=CARTESIAN_POINT ( 'NONE',  ( 1.467888652718972731, -5.050659073900638063, 3.492485675378566246 ) ) ;
#1462=AXIS2_PLACEMENT_3D ( 'NONE', #3623, #6446, #2975 ) ;
#1474=CARTESIAN_POINT ( 'NONE',  ( -3.007514324621463508, -5.149340926099361226, 1.224499502706077658 ) ) ;
#1477=CARTESIAN_POINT ( 'NONE',  ( -4.007514324621431534, -7.650659073900639484, -1.638713065079248521 ) ) ;
#1486=CARTESIAN_POINT ( 'NONE',  ( -2.108492589042306964, -6.449340926099361049, -2.134148098076978251 ) ) ;
#1500=CARTESIAN_POINT ( 'NONE',  ( -3.500000000000000000, -6.649340926099361226, -0.01814118441321344033 ) ) ;
#1510=CARTESIAN_POINT ( 'NONE',  ( -0.01814118441313947866, -4.150659073900639484, -3.500000000000000000 ) ) ;
#1518=CARTESIAN_POINT ( 'NONE',  ( 2.487701488670255756, -1.249340926099361093, -2.462045979635577364 ) ) ;
#1520=CARTESIAN_POINT ( 'NONE',  ( -1.260781871532494103, -2.149340926099361226, 2.992485675378538712 ) ) ;
#1523=CARTESIAN_POINT ( 'NONE',  ( -0.01814118441313417734, -7.350659073900637885, -4.000000000000000000 ) ) ;
#1534=CARTESIAN_POINT ( 'NONE',  ( -2.108492589042352261, -3.150659073900639484, 2.134148098076933397 ) ) ;
#1545=CARTESIAN_POINT ( 'NONE',  ( -1.467888652719046449, -2.149340926099360782, 3.492485675378536047 ) ) ;
#1548=CARTESIAN_POINT ( 'NONE',  ( -2.487701488670255312, -6.849340926099361404, 2.462045979635577808 ) ) ;
#1551=CARTESIAN_POINT ( 'NONE',  ( -0.01814118441313947866, -7.350659073900638774, -3.500000000000000000 ) ) ;
#1558=CARTESIAN_POINT ( 'NONE',  ( -2.841254879263473310, -5.950659073900640195, -2.815599370228907716 ) ) ;
#1565=CARTESIAN_POINT ( 'NONE',  ( 1.467888652719048226, -2.949340926099361493, -3.492485675378536047 ) ) ;
#1568=CARTESIAN_POINT ( 'NONE',  ( 2.108492589042352705, -0.7506590739006395729, -2.134148098076933397 ) ) ;
#1570=CARTESIAN_POINT ( 'NONE',  ( 3.992485675378533383, -0.9493409260993608267, 1.674995433905599462 ) ) ;
#1582=CARTESIAN_POINT ( 'NONE',  ( -1.224499502706140497, -3.250659073900639573, 3.007514324621436863 ) ) ;
#1589=CARTESIAN_POINT ( 'NONE',  ( -3.492485675378536047, -6.549340926099363358, -1.467888652719048670 ) ) ;
#1594=ORIENTED_EDGE ( 'NONE', *, *, #3658, .F. ) ;
#1601=CARTESIAN_POINT ( 'NONE',  ( 3.992485675378568910, -3.850659073900639662, -1.674995433905514863 ) ) ;
#1607=EDGE_CURVE ( 'NONE', #183, #2600, #6516, .T. ) ;
#1613=CARTESIAN_POINT ( 'NONE',  ( 1.260781871532430598, -5.050659073900640728, 2.992485675378564469 ) ) ;
#1616=CARTESIAN_POINT ( 'NONE',  ( 2.841254879263473310, -6.750659073900638241, 2.815599370228907272 ) ) ;
#1621=CARTESIAN_POINT ( 'NONE',  ( 1.467888652719048226, -1.349340926099361182, -3.492485675378535603 ) ) ;
#1625=CARTESIAN_POINT ( 'NONE',  ( 4.007514324621469726, -2.749340926099360427, -1.638713065079161257 ) ) ;
#1630=CARTESIAN_POINT ( 'NONE',  ( 1.467888652718972731, -0.2506590739006389068, 3.492485675378566246 ) ) ;
#1640=CARTESIAN_POINT ( 'NONE',  ( 3.492485675378536047, -0.9493409260993610488, 1.467888652719046672 ) ) ;
#1654=CARTESIAN_POINT ( 'NONE',  ( -2.815599370228907272, -4.750659073900638241, 2.841254879263473754 ) ) ;
#1664=CARTESIAN_POINT ( 'NONE',  ( -3.007514324621435531, -4.450659073900640195, -1.224499502706142273 ) ) ;
#1666=CARTESIAN_POINT ( 'NONE',  ( -3.992485675378532939, -3.349340926099360960, -1.674995433905601683 ) ) ;
#1669=CARTESIAN_POINT ( 'NONE',  ( 3.507514324621465285, -5.949340926099361049, -1.431606283892619347 ) ) ;
#1673=CARTESIAN_POINT ( 'NONE',  ( -4.000000000000000000, -5.049340926099361582, -0.01814118441321865144 ) ) ;
#1677=CARTESIAN_POINT ( 'NONE',  ( -0.01814118441313947866, -0.9506590739006390844, -3.500000000000000000 ) ) ;
#1686=ADVANCED_FACE ( 'NONE', ( #7882 ), #5347, .T. ) ;
#1688=CARTESIAN_POINT ( 'NONE',  ( 2.487701488670255756, -4.449340926099361937, -2.462045979635577364 ) ) ;
#1697=SHAPE_REPRESENTATION ( 'spring', ( #888 ), #3388 ) ;
#1701=CARTESIAN_POINT ( 'NONE',  ( 3.992485675378568910, -7.050659073900638063, -1.674995433905514863 ) ) ;
#1711=CARTESIAN_POINT ( 'NONE',  ( 1.260781871532430598, -3.450659073900639751, 2.992485675378564469 ) ) ;
#1715=CARTESIAN_POINT ( 'NONE',  ( 0.01814118441321408565, -3.049340926099361138, -3.500000000000000000 ) ) ;
#1722=CARTESIAN_POINT ( 'NONE',  ( 3.992485675378533383, -5.749340926099361759, 1.674995433905599462 ) ) ;
#1726=CARTESIAN_POINT ( 'NONE',  ( -0.01814118441314477650, -5.750659073900639129, -3.000000000000000444 ) ) ;
#1729=CARTESIAN_POINT ( 'NONE',  ( 3.500000000000000000, -2.150659073900639040, -0.01814118441313969030 ) ) ;
#1736=CARTESIAN_POINT ( 'NONE',  ( 1.431606283892619125, -2.349340926099361848, 3.507514324621464397 ) ) ;
#1748=CARTESIAN_POINT ( 'NONE',  ( -2.841254879263473310, -7.550659073900639839, -2.815599370228907716 ) ) ;
#1759=CARTESIAN_POINT ( 'NONE',  ( 2.134148098076933397, -5.150659073900639484, 2.108492589042352261 ) ) ;
#1765=CARTESIAN_POINT ( 'NONE',  ( 0.01814118441321408565, -4.649340926099361226, -3.500000000000000000 ) ) ;
#1770=CARTESIAN_POINT ( 'NONE',  ( 1.674995433905601239, -7.749340926099362648, -3.992485675378532939 ) ) ;
#1774=CARTESIAN_POINT ( 'NONE',  ( -2.487701488670202910, -4.350659073900638774, -2.462045979635629767 ) ) ;
#1778=CARTESIAN_POINT ( 'NONE',  ( -3.492485675378566246, -3.050659073900638951, 1.467888652718973175 ) ) ;
#1785=CARTESIAN_POINT ( 'NONE',  ( -1.260781871532494103, -3.749340926099361315, 2.992485675378538712 ) ) ;
#1791=CARTESIAN_POINT ( 'NONE',  ( -2.007298707674168181, -4.858300672349188093E-16, 2.776755344285330107 ) ) ;
#1809=CARTESIAN_POINT ( 'NONE',  ( -3.492485675378566246, -1.450659073900639084, 1.467888652718973397 ) ) ;
#1813=CARTESIAN_POINT ( 'NONE',  ( 3.507514324621465285, -1.149340926099361226, -1.431606283892619347 ) ) ;
#1818=CARTESIAN_POINT ( 'NONE',  ( 2.841254879263533262, -6.049340926099361582, -2.815599370228847320 ) ) ;
#1821=CARTESIAN_POINT ( 'NONE',  ( -3.507514324621434199, -4.450659073900639306, -1.431606283892695064 ) ) ;
#1825=CARTESIAN_POINT ( 'NONE',  ( -1.925759277493323207, -9.035843541029836168E-14, 2.922632427747480222 ) ) ;
#1831=APPLICATION_CONTEXT ( 'automotive_design' ) ;
#1833=CARTESIAN_POINT ( 'NONE',  ( -2.108492589042306964, -1.649340926099361448, -2.134148098076978251 ) ) ;
#1845=VECTOR ( 'NONE', #5986, 1000.000000000000000 ) ;
#1852=CARTESIAN_POINT ( 'NONE',  ( 0.01814118441321408565, -3.049340926099361138, -3.500000000000000000 ) ) ;
#1858=EDGE_LOOP ( 'NONE', ( #6387, #8496, #2011, #9019, #5652 ) ) ;
#1861=CARTESIAN_POINT ( 'NONE',  ( -3.000000000000000444, -7.750659073900639129, 0.01814118441314532468 ) ) ;
#1872=CARTESIAN_POINT ( 'NONE',  ( 0.01814118441321408565, -4.649340926099361226, -3.500000000000000000 ) ) ;
#1875=CARTESIAN_POINT ( 'NONE',  ( -2.462045979635629323, -3.150659073900639040, 2.487701488670203798 ) ) ;
#1885=CARTESIAN_POINT ( 'NONE',  ( 1.467888652719048226, -7.749340926099361759, -3.492485675378536047 ) ) ;
#1896=CARTESIAN_POINT ( 'NONE',  ( 1.638713065079161924, -7.149340926099361226, 4.007514324621467949 ) ) ;
#1903=CARTESIAN_POINT ( 'NONE',  ( 0.01814118441313990887, -0.1506590739006389568, 3.500000000000000000 ) ) ;
#1914=CARTESIAN_POINT ( 'NONE',  ( -3.507514324621464397, -3.549340926099361582, 1.431606283892619347 ) ) ;
#1918=CARTESIAN_POINT ( 'NONE',  ( 3.507514324621434199, -3.650659073900639928, 1.431606283892693066 ) ) ;
#1922=CARTESIAN_POINT ( 'NONE',  ( -2.462045979635629323, -4.750659073900639129, 2.487701488670203798 ) ) ;
#1928=CARTESIAN_POINT ( 'NONE',  ( 2.992485675378538712, -2.549340926099361582, 1.260781871532494103 ) ) ;
#1940=CARTESIAN_POINT ( 'NONE',  ( -3.500000000000000000, -0.2493409260993610654, -0.01814118441321344033 ) ) ;
#1942=CARTESIAN_POINT ( 'NONE',  ( 1.467888652719048226, -2.949340926099361493, -3.492485675378536047 ) ) ;
#1949=CARTESIAN_POINT ( 'NONE',  ( -3.507514324621434199, -1.250659073900638907, -1.431606283892695064 ) ) ;
#1951=CIRCLE ( 'NONE', #295, 0.2499999999999998335 ) ;
#1961=CARTESIAN_POINT ( 'NONE',  ( 3.500000000000000000, -4.249340926099360871, 0.01814118441321387054 ) ) ;
#1964=CARTESIAN_POINT ( 'NONE',  ( 3.492485675378566690, -3.850659073900639218, -1.467888652718972287 ) ) ;
#1970=CARTESIAN_POINT ( 'NONE',  ( -3.007514324621463508, -1.949340926099361493, 1.224499502706077658 ) ) ;
#1980=CARTESIAN_POINT ( 'NONE',  ( -3.431411822166540393, -3.932028342760356289E-17, 1.490417237447617449 ) ) ;
#1982=CARTESIAN_POINT ( 'NONE',  ( -1.638713065079163034, -7.949340926099362825, -4.007514324621466173 ) ) ;
#1983=CARTESIAN_POINT ( 'NONE',  ( -3.507514324621464397, -0.3493409260993610710, 1.431606283892619347 ) ) ;
#1994=CARTESIAN_POINT ( 'NONE',  ( -1.467888652718973619, -2.650659073900639040, -3.492485675378565801 ) ) ;
#1999=CARTESIAN_POINT ( 'NONE',  ( -1.467888652719046449, -6.949340926099361049, 3.492485675378535603 ) ) ;
#2004=CARTESIAN_POINT ( 'NONE',  ( -1.431606283892620235, -7.949340926099361049, -3.507514324621463953 ) ) ;
#2008=CARTESIAN_POINT ( 'NONE',  ( -3.992485675378568022, -1.450659073900638862, 1.674995433905515529 ) ) ;
#2011=ORIENTED_EDGE ( 'NONE', *, *, #872, .T. ) ;
#2015=CARTESIAN_POINT ( 'NONE',  ( 2.108492589042307408, -5.649340926099361226, 2.134148098076978251 ) ) ;
#2028=CARTESIAN_POINT ( 'NONE',  ( 2.487701488670255756, -4.449340926099361937, -2.462045979635577364 ) ) ;
#2029=CARTESIAN_POINT ( 'NONE',  ( -4.000000000000000000, -8.249340926099360871, -0.01814118441321865144 ) ) ;
#2036=CARTESIAN_POINT ( 'NONE',  ( -3.507514324621434199, -7.650659073900639484, -1.431606283892695064 ) ) ;
#2045=CARTESIAN_POINT ( 'NONE',  ( -3.000000000000000444, -6.649340926099362115, -0.01814118441320822922 ) ) ;
#2049=CARTESIAN_POINT ( 'NONE',  ( -0.01814118441313417734, -4.150659073900638596, -4.000000000000000000 ) ) ;
#2052=CARTESIAN_POINT ( 'NONE',  ( -1.922037972912167048, -5.459919674189117688E-16, 2.905699108924820084 ) ) ;
#2057=CARTESIAN_POINT ( 'NONE',  ( -3.000000000000000444, -2.950659073900639306, 0.01814118441314532468 ) ) ;
#2066=CARTESIAN_POINT ( 'NONE',  ( -1.431606283892620235, -4.749340926099363536, -3.507514324621463953 ) ) ;
#2067=CARTESIAN_POINT ( 'NONE',  ( -1.467888652719046449, -5.349340926099361404, 3.492485675378536047 ) ) ;
#2077=CARTESIAN_POINT ( 'NONE',  ( -3.992485675378568022, -1.450659073900638862, 1.674995433905515529 ) ) ;
#2091=CARTESIAN_POINT ( 'NONE',  ( 2.992485675378538712, -5.749340926099361759, 1.260781871532494103 ) ) ;
#2094=CARTESIAN_POINT ( 'NONE',  ( 3.992485675378568910, -3.850659073900639662, -1.674995433905514863 ) ) ;
#2102=CARTESIAN_POINT ( 'NONE',  ( 2.992485675378538712, -7.349340926099363180, 1.260781871532494103 ) ) ;
#2112=CARTESIAN_POINT ( 'NONE',  ( -1.467888652719046449, -2.149340926099360782, 3.492485675378536047 ) ) ;
#2113=CARTESIAN_POINT ( 'NONE',  ( -3.492485675378536047, -3.349340926099361404, -1.467888652719048670 ) ) ;
#2120=CARTESIAN_POINT ( 'NONE',  ( -1.638713065079245634, -1.650659073900638818, 4.007514324621432422 ) ) ;
#2133=CARTESIAN_POINT ( 'NONE',  ( -3.007514324621463508, -3.549340926099361582, 1.224499502706077658 ) ) ;
#2137=CARTESIAN_POINT ( 'NONE',  ( 2.841254879263473310, -5.150659073900639484, 2.815599370228907272 ) ) ;
#2147=CARTESIAN_POINT ( 'NONE',  ( -2.134148098076978251, -6.849340926099361404, 2.108492589042307408 ) ) ;
#2152=( LENGTH_UNIT ( ) NAMED_UNIT ( * ) SI_UNIT ( .MILLI., .METRE. ) );
#2158=CARTESIAN_POINT ( 'NONE',  ( 3.492485675378536047, -7.349340926099362292, 1.467888652719046672 ) ) ;
#2159=CARTESIAN_POINT ( 'NONE',  ( 0.01814118441321408565, -7.849340926099360516, -3.500000000000000000 ) ) ;
#2166=CARTESIAN_POINT ( 'NONE',  ( -3.500000000000000000, -4.550659073900638951, 0.01814118441314012051 ) ) ;
#2176=CARTESIAN_POINT ( 'NONE',  ( -1.224499502706077880, -3.149340926099362115, -3.007514324621463064 ) ) ;
#2179=CARTESIAN_POINT ( 'NONE',  ( -2.815599370228907272, -6.350659073900638774, 2.841254879263473754 ) ) ;
#2183=EDGE_LOOP ( 'NONE', ( #7881, #4303, #254 ) ) ;
#2187=CARTESIAN_POINT ( 'NONE',  ( 3.007514324621436863, -2.050659073900639839, 1.224499502706140719 ) ) ;
#2191=PRODUCT_DEFINITION_FORMATION_WITH_SPECIFIED_SOURCE ( 'ANY', '', #4156, .NOT_KNOWN. ) ;
#2194=SURFACE_SIDE_STYLE ('',( #8483 ) ) ;
#2201=CARTESIAN_POINT ( 'NONE',  ( 3.500000000000000000, -5.849340926099361404, 0.01814118441321387054 ) ) ;
#2203=CARTESIAN_POINT ( 'NONE',  ( -3.500000000000000000, 0.2493409260993610654, 0.01814118441314012051 ) ) ;
#2206=EDGE_LOOP ( 'NONE', ( #5156, #2359, #139 ) ) ;
#2210=CARTESIAN_POINT ( 'NONE',  ( -1.674995433905516196, -1.050659073900638507, -3.992485675378566690 ) ) ;
#2220=CARTESIAN_POINT ( 'NONE',  ( -3.007514324621463508, -6.749340926099361759, 1.224499502706077658 ) ) ;
#2224=CARTESIAN_POINT ( 'NONE',  ( -4.007514324621467949, -0.3493409260993607379, 1.638713065079161924 ) ) ;
#2234=CARTESIAN_POINT ( 'NONE',  ( -2.992485675378564469, -4.650659073900640372, 1.260781871532430820 ) ) ;
#2242=FILL_AREA_STYLE ('',( #8565 ) ) ;
#2244=CARTESIAN_POINT ( 'NONE',  ( -3.492485675378536047, -1.749340926099361093, -1.467888652719048670 ) ) ;
#2248=CARTESIAN_POINT ( 'NONE',  ( -0.01814118441321365544, -5.449340926099361937, 3.500000000000000000 ) ) ;
#2258=CARTESIAN_POINT ( 'NONE',  ( -2.841254879263533262, -0.4493409260993607157, 2.815599370228847764 ) ) ;
#2266=CARTESIAN_POINT ( 'NONE',  ( 3.500000000000000000, -2.649340926099361226, 0.01814118441321387054 ) ) ;
#2268=CARTESIAN_POINT ( 'NONE',  ( 3.007514324621436863, -3.650659073900639928, 1.224499502706140719 ) ) ;
#2270=CARTESIAN_POINT ( 'NONE',  ( -0.01814118441321889430, -2.249340926099360427, 4.000000000000000000 ) ) ;
#2283=CARTESIAN_POINT ( 'NONE',  ( 3.000000000000000444, -5.350659073900639662, -0.01814118441314496039 ) ) ;
#2288=( NAMED_UNIT ( * ) PLANE_ANGLE_UNIT ( ) SI_UNIT ( $, .RADIAN. ) );
#2292=CARTESIAN_POINT ( 'NONE',  ( 0.01814118441321408565, -6.249340926099360871, -3.500000000000000000 ) ) ;
#2299=CARTESIAN_POINT ( 'NONE',  ( 0.01814118441313990887, -6.550659073900639839, 3.500000000000000000 ) ) ;
#2307=CARTESIAN_POINT ( 'NONE',  ( -2.841254879263473310, -4.350659073900638774, -2.815599370228907716 ) ) ;
#2314=CARTESIAN_POINT ( 'NONE',  ( -1.467888652719046449, -0.5493409260993611376, 3.492485675378536047 ) ) ;
#2316=CARTESIAN_POINT ( 'NONE',  ( 3.000000000000000444, -3.750659073900639573, -0.01814118441314496039 ) ) ;
#2318=CARTESIAN_POINT ( 'NONE',  ( 4.000000000000000000, -6.950659073900639306, -0.01814118441313441674 ) ) ;
#2326=CARTESIAN_POINT ( 'NONE',  ( -2.841254879263533262, -5.249340926099361759, 2.815599370228847764 ) ) ;
#2330=CARTESIAN_POINT ( 'NONE',  ( 0.01814118441313990887, -0.1506590739006389568, 3.500000000000000000 ) ) ;
#2336=CARTESIAN_POINT ( 'NONE',  ( 3.500000000000000000, -4.249340926099360871, 0.01814118441321387054 ) ) ;
#2343=DIRECTION ( 'NONE',  ( 1.044949058366721163E-14, 0.07256473765270718412, -0.9973637043974449279 ) ) ;
#2350=CARTESIAN_POINT ( 'NONE',  ( -4.000000000000000000, -2.950659073900638862, 0.01814118441313491634 ) ) ;
#2359=ORIENTED_EDGE ( 'NONE', *, *, #885, .F. ) ;
#2362=CARTESIAN_POINT ( 'NONE',  ( -1.260781871532431708, -4.250659073900640017, -2.992485675378564469 ) ) ;
#2364=CARTESIAN_POINT ( 'NONE',  ( 2.841254879263533262, -1.249340926099360871, -2.815599370228847320 ) ) ;
#2368=CARTESIAN_POINT ( 'NONE',  ( -3.507514324621464397, -1.949340926099361271, 1.431606283892619569 ) ) ;
#2374=CARTESIAN_POINT ( 'NONE',  ( -2.841254879263533262, -3.649340926099360782, 2.815599370228847764 ) ) ;
#2378=CARTESIAN_POINT ( 'NONE',  ( -3.007514324621435531, -7.650659073900639484, -1.224499502706142273 ) ) ;
#2386=CARTESIAN_POINT ( 'NONE',  ( 3.492485675378536047, -2.549340926099360694, 1.467888652719046672 ) ) ;
#2398=CARTESIAN_POINT ( 'NONE',  ( 1.674995433905515085, -6.650659073900639484, 3.992485675378568022 ) ) ;
#2408=CARTESIAN_POINT ( 'NONE',  ( -1.224499502706140497, -3.250659073900639573, 3.007514324621436863 ) ) ;
#2413=CARTESIAN_POINT ( 'NONE',  ( -1.467888652719046449, -0.5493409260993611376, 3.492485675378535603 ) ) ;
#2419=CARTESIAN_POINT ( 'NONE',  ( 3.992485675378533383, -7.349340926099363180, 1.674995433905599462 ) ) ;
#2423=CARTESIAN_POINT ( 'NONE',  ( -1.431606283892693066, -0.05065907390063895815, 3.507514324621434199 ) ) ;
#2436=CARTESIAN_POINT ( 'NONE',  ( 2.462045979635577364, -0.8493409260993610710, 2.487701488670255312 ) ) ;
#2449=CARTESIAN_POINT ( 'NONE',  ( 1.638713065079247855, -7.250659073900640017, -4.007514324621431534 ) ) ;
#2459=CARTESIAN_POINT ( 'NONE',  ( 2.992485675378565357, -0.6506590739006395951, -1.260781871532430376 ) ) ;
#2463=CARTESIAN_POINT ( 'NONE',  ( -3.507514324621464397, -5.149340926099361226, 1.431606283892619569 ) ) ;
#2468=CARTESIAN_POINT ( 'NONE',  ( -0.01814118441321889430, -3.849340926099360960, 4.000000000000000000 ) ) ;
#2472=CARTESIAN_POINT ( 'NONE',  ( 3.507514324621434199, -2.050659073900638951, 1.431606283892693066 ) ) ;
#2476=CARTESIAN_POINT ( 'NONE',  ( -3.507514324621433754, -2.850659073900639218, -1.431606283892695064 ) ) ;
#2482=CARTESIAN_POINT ( 'NONE',  ( 3.007514324621463508, -2.749340926099361759, -1.224499502706076770 ) ) ;
#2503=CARTESIAN_POINT ( 'NONE',  ( 1.431606283892694842, -0.8506590739006389956, -3.507514324621434199 ) ) ;
#2507=CARTESIAN_POINT ( 'NONE',  ( 3.500000000000000000, -5.849340926099361404, 0.01814118441321387054 ) ) ;
#2514=CARTESIAN_POINT ( 'NONE',  ( -2.841254879263533262, -2.049340926099361138, 2.815599370228847764 ) ) ;
#2517=CARTESIAN_POINT ( 'NONE',  ( 0.01814118441313990887, -3.350659073900639218, 3.500000000000000000 ) ) ;
#2522=CARTESIAN_POINT ( 'NONE',  ( -2.487701488670202910, -7.550659073900639839, -2.462045979635629767 ) ) ;
#2525=STYLED_ITEM('',(#9225),#8451);
#2529=CARTESIAN_POINT ( 'NONE',  ( 2.108492589042307408, -0.8493409260993616261, 2.134148098076978251 ) ) ;
#2546=CARTESIAN_POINT ( 'NONE',  ( 2.487701488670255756, -1.249340926099361093, -2.462045979635577364 ) ) ;
#2557=CARTESIAN_POINT ( 'NONE',  ( 3.000000000000000444, -6.950659073900640195, -0.01814118441314496039 ) ) ;
#2569=CARTESIAN_POINT ( 'NONE',  ( -2.462045979635576920, -8.049340926099361582, -2.487701488670255756 ) ) ;
#2573=CARTESIAN_POINT ( 'NONE',  ( -2.487701488670202910, -7.550659073900639839, -2.462045979635629767 ) ) ;
#2576=CARTESIAN_POINT ( 'NONE',  ( -1.431606283892693066, -1.650659073900639040, 3.507514324621434199 ) ) ;
#2582=CARTESIAN_POINT ( 'NONE',  ( -3.492485675378536047, -8.149340926099361226, -1.467888652719048670 ) ) ;
#2599=CARTESIAN_POINT ( 'NONE',  ( -1.431606283892620235, -3.149340926099361671, -3.507514324621463953 ) ) ;
#2600=VERTEX_POINT ( 'NONE', #8678 ) ;
#2608=CARTESIAN_POINT ( 'NONE',  ( -3.507514324621434199, -2.850659073900639662, -1.431606283892695064 ) ) ;
#2618=CARTESIAN_POINT ( 'NONE',  ( 0.01814118441321408565, -3.049340926099361138, -3.500000000000000000 ) ) ;
#2621=CARTESIAN_POINT ( 'NONE',  ( -2.487701488670202910, -2.750659073900639129, -2.462045979635629767 ) ) ;
#2625=CARTESIAN_POINT ( 'NONE',  ( 3.507514324621434199, -0.4506590739006389734, 1.431606283892693066 ) ) ;
#2631=CARTESIAN_POINT ( 'NONE',  ( 3.507514324621465285, -7.549340926099362470, -1.431606283892619125 ) ) ;
#2642=CARTESIAN_POINT ( 'NONE',  ( -3.492485675378536047, -4.949340926099361049, -1.467888652719048670 ) ) ;
#2643=CARTESIAN_POINT ( 'NONE',  ( -3.500000000000000000, -1.849340926099361182, -0.01814118441321344033 ) ) ;
#2650=CARTESIAN_POINT ( 'NONE',  ( 3.500000000000000000, -3.750659073900639129, -0.01814118441313969030 ) ) ;
#2660=CARTESIAN_POINT ( 'NONE',  ( -3.500000000000000000, -3.449340926099361049, -0.01814118441321344033 ) ) ;
#2664=CARTESIAN_POINT ( 'NONE',  ( 2.487701488670203354, -1.950659073900639084, 2.462045979635629323 ) ) ;
#2668=CARTESIAN_POINT ( 'NONE',  ( -3.507514324621433754, -4.450659073900639306, -1.431606283892695064 ) ) ;
#2673=CARTESIAN_POINT ( 'NONE',  ( 1.224499502706077214, -0.7493409260993615373, 3.007514324621463508 ) ) ;
#2684=CARTESIAN_POINT ( 'NONE',  ( -3.500000000000000000, -1.849340926099361182, -0.01814118441321344033 ) ) ;
#2687=CARTESIAN_POINT ( 'NONE',  ( 0.01814118441321408565, -1.449340926099361271, -3.500000000000000000 ) ) ;
#2695=CARTESIAN_POINT ( 'NONE',  ( 3.007514324621436863, -6.850659073900641438, 1.224499502706140719 ) ) ;
#2700=CARTESIAN_POINT ( 'NONE',  ( -0.01814118441321365544, -7.049340926099361582, 3.500000000000000000 ) ) ;
#2704=CARTESIAN_POINT ( 'NONE',  ( -3.500000000000000000, -5.049340926099361582, -0.01814118441321344033 ) ) ;
#2708=CARTESIAN_POINT ( 'NONE',  ( 2.815599370228907716, -5.550659073900638063, -2.841254879263473310 ) ) ;
#2718=CARTESIAN_POINT ( 'NONE',  ( 2.992485675378538712, -5.749340926099361759, 1.260781871532494103 ) ) ;
#2729=CARTESIAN_POINT ( 'NONE',  ( -3.492485675378536047, -3.349340926099361404, -1.467888652719048670 ) ) ;
#2730=CARTESIAN_POINT ( 'NONE',  ( 1.674995433905601239, -7.749340926099362648, -3.992485675378532939 ) ) ;
#2744=CARTESIAN_POINT ( 'NONE',  ( -0.01814118441313947866, -5.750659073900639129, -3.500000000000000000 ) ) ;
#2748=CARTESIAN_POINT ( 'NONE',  ( 1.467888652719048226, -6.149340926099361226, -3.492485675378535603 ) ) ;
#2752=CARTESIAN_POINT ( 'NONE',  ( 1.224499502706077214, -0.7493409260993615373, 3.007514324621463508 ) ) ;
#2756=CARTESIAN_POINT ( 'NONE',  ( 4.000000000000000000, -0.5506590739006383961, -0.01814118441313441674 ) ) ;
#2765=CARTESIAN_POINT ( 'NONE',  ( -0.01814118441320841310, -5.449340926099361937, 3.000000000000000444 ) ) ;
#2776=CARTESIAN_POINT ( 'NONE',  ( -2.462045979635576920, -4.849340926099361404, -2.487701488670255756 ) ) ;
#2777=CARTESIAN_POINT ( 'NONE',  ( -2.487701488670255312, -6.849340926099361404, 2.462045979635577808 ) ) ;
#2785=CARTESIAN_POINT ( 'NONE',  ( 0.01814118441313467001, -0.1506590739006384849, 4.000000000000000000 ) ) ;
#2796=CARTESIAN_POINT ( 'NONE',  ( 1.224499502706077214, -5.549340926099361582, 3.007514324621463508 ) ) ;
#2798=( GEOMETRIC_REPRESENTATION_CONTEXT ( 3 ) GLOBAL_UNCERTAINTY_ASSIGNED_CONTEXT ( ( #3022 ) ) GLOBAL_UNIT_ASSIGNED_CONTEXT ( ( #2152, #748, #6508 ) ) REPRESENTATION_CONTEXT ( 'NONE', 'WORKASPACE' ) );
#2800=CARTESIAN_POINT ( 'NONE',  ( -2.815599370228907272, -3.150659073900639040, 2.841254879263473754 ) ) ;
#2808=CARTESIAN_POINT ( 'NONE',  ( -2.992485675378564469, -3.050659073900639839, 1.260781871532430820 ) ) ;
#2820=CARTESIAN_POINT ( 'NONE',  ( -0.01814118441321365544, -5.449340926099361937, 3.500000000000000000 ) ) ;
#2831=CARTESIAN_POINT ( 'NONE',  ( 2.462045979635629767, -7.150659073900639484, -2.487701488670203354 ) ) ;
#2842=CARTESIAN_POINT ( 'NONE',  ( 2.108492589042307408, -7.249340926099360871, 2.134148098076978251 ) ) ;
#2846=CARTESIAN_POINT ( 'NONE',  ( -1.674995433905516196, -1.050659073900638507, -3.992485675378566690 ) ) ;
#2856=CARTESIAN_POINT ( 'NONE',  ( -1.260781871532494103, -6.949340926099362825, 2.992485675378538712 ) ) ;
#2863=CARTESIAN_POINT ( 'NONE',  ( -2.475000949148032703, -1.535234168964353515E-16, 2.672592990517839606 ) ) ;
#2866=CARTESIAN_POINT ( 'NONE',  ( -3.507514324621464397, -3.549340926099361582, 1.431606283892619347 ) ) ;
#2873=CARTESIAN_POINT ( 'NONE',  ( 1.431606283892694842, -7.250659073900640017, -3.507514324621434199 ) ) ;
#2887=CARTESIAN_POINT ( 'NONE',  ( -3.000000000000000444, -3.449340926099361493, -0.01814118441320822922 ) ) ;
#2890=CARTESIAN_POINT ( 'NONE',  ( -1.674995433905516196, -2.650659073900639040, -3.992485675378566690 ) ) ;
#2898=CARTESIAN_POINT ( 'NONE',  ( 2.134148098076933397, -1.950659073900639306, 2.108492589042352261 ) ) ;
#2910=CARTESIAN_POINT ( 'NONE',  ( -3.492485675378536047, -8.149340926099361226, -1.467888652719048670 ) ) ;
#2911=CARTESIAN_POINT ( 'NONE',  ( 1.431606283892619125, -7.149340926099362115, 3.507514324621464397 ) ) ;
#2913=CARTESIAN_POINT ( 'NONE',  ( -3.507514324621433754, -6.050659073900638951, -1.431606283892695064 ) ) ;
#2920=CARTESIAN_POINT ( 'NONE',  ( 2.841254879263473310, -0.3506590739006385515, 2.815599370228907272 ) ) ;
#2929=CARTESIAN_POINT ( 'NONE',  ( 0.01814118441320878086, -6.249340926099361759, -3.000000000000000444 ) ) ;
#2932=CARTESIAN_POINT ( 'NONE',  ( 4.007514324621469726, -2.749340926099360427, -1.638713065079161257 ) ) ;
#2940=CARTESIAN_POINT ( 'NONE',  ( -3.500000000000000000, -1.350659073900638996, 0.01814118441314012051 ) ) ;
#2950=( BOUNDED_SURFACE ( )  B_SPLINE_SURFACE ( 3, 2, ( 
 ( #1319, #6996, #622, #3464, #5216, #5913, #2436, #1640, #4528, #3142, #3829, #195, #7216, #4477, #5262, #2244, #7315, #8800, #285, #1545, #5866, #1736, #6703, #2386, #840, #8058, #4386, #6655, #3090, #7359, #6611, #983, #940, #3048, #892, #240, #8706, #5962, #7920, #5067, #2336, #3687, #1688, #8755, #8107, #3788, #4572, #7408, #1031, #5167, #6512, #3881, #332, #149, #3185, #8613, #2999, #5821, #8009, #8660, #2292, #5117, #7964, #1589, #4429, #7264, #3742, #6563, #477, #6199, #527, #6854, #1270, #2631, #1132, #1885, #380, #6754, #6801, #2582, #3368 ),
 ( #3273, #8203, #4619, #426, #569, #2673, #2529, #9027, #7458, #4756, #3926, #5498, #8345, #5306, #1833, #4665, #5402, #1970, #3229, #6940, #5450, #6154, #4710, #1928, #4799, #2482, #8888, #1176, #8252, #7504, #5354, #3972, #6050, #8295, #4019, #1785, #7642, #6103, #7600, #1224, #4064, #7549, #6006, #8933, #3323, #4108, #8845, #1084, #8982, #6903, #8157, #4241, #2765, #7031, #2015, #2718, #4840, #5716, #4151, #7072, #696, #614, #1486, #1357, #3455, #4330, #2147, #2856, #4968, #3541, #658, #2102, #7822, #4925, #4196, #4882, #1400, #3500, #1438, #5543, #9076 ),
 ( #6366, #6411, #5628, #8520, #7117, #4284, #6323, #7685, #8477, #50, #6242, #7778, #3587, #740, #8388, #9159, #8559, #7163, #5, #1309, #5672, #6986, #2898, #2187, #5009, #7865, #3413, #6284, #9120, #5585, #8429, #7733, #2057, #2808, #1534, #1582, #6555, #7350, #7912, #5813, #4563, #7255, #2989, #8603, #4423, #790, #6647, #6501, #4521, #2234, #8744, #4377, #276, #976, #90, #8651, #2283, #185, #3130, #7209, #1726, #234, #929, #5859, #5905, #5953, #6456, #3679, #5159, #3040, #5109, #138, #7958, #834, #3083, #8001, #5761, #8792, #882, #2378, #5207 ),
 ( #8699, #3731, #5059, #2423, #2330, #1630, #4468, #7306, #3779, #6605, #3634, #8049, #1677, #3822, #5253, #8098, #2940, #6190, #4610, #3311, #7398, #3219, #2664, #2472, #6842, #6143, #7538, #4652, #6090, #8971, #2621, #6039, #5438, #8876, #1875, #8284, #2517, #5486, #518, #1918, #8334, #1964, #466, #4742, #5343, #8192, #1774, #1821, #7589, #6741, #1073, #3360, #1021, #1215, #3962, #4699, #3175, #3916, #5997, #371, #3871, #4055, #1164, #6692, #8147, #7495, #5296, #1121, #322, #9018, #7448, #6890, #6788, #414, #4008, #8836, #3262, #8923, #2573, #5390, #8241 ),
 ( #8421, #7814, #7767, #8511, #1390, #3534, #4919, #5619, #2756, #9067, #4143, #731, #1431, #2846, #1301, #7721, #4234, #2008, #5707, #7108, #7064, #6404, #4276, #9152, #3449, #3579, #562, #40, #688, #2890, #6976, #6358, #6316, #6276, #2800, #1349, #3491, #6235, #7634, #9111, #8466, #2094, #5577, #3401, #2049, #646, #7020, #4874, #3406, #8551, #605, #4187, #5665, #5536, #2137, #4959, #1262, #4790, #2708, #4102, #6934, #8379, #4833, #7679, #8594, #7293, #2179, #7201, #6767, #6448, #1616, #917, #2318, #8639, #866, #3765, #1523, #5801, #779, #1477, #3626 ),
 ( #3024, #2224, #395, #127, #5049, #3242, #6593, #1570, #7156, #4507, #2364, #223, #82, #3072, #174, #5893, #3716, #2976, #3668, #5847, #2270, #8733, #4320, #7857, #5098, #2932, #7987, #8687, #5194, #4411, #8036, #1666, #7338, #7948, #5753, #7242, #1100, #5000, #6542, #3940, #6066, #7904, #5146, #4367, #825, #4454, #6493, #8358, #4679, #6954, #3381, #4770, #6214, #9089, #3428, #540, #4166, #5515, #4035, #7614, #3290, #444, #493, #5464, #6257, #6817, #4723, #3468, #6169, #1896, #7516, #3340, #8901, #5557, #5416, #2730, #1145, #7659, #6118, #8401, #2029 ),
 ( #4852, #1983, #1323, #7698, #4080, #7564, #7000, #3988, #626, #4814, #2546, #8265, #2687, #1238, #1192, #6916, #2643, #9043, #8947, #5369, #6869, #1281, #4120, #8995, #584, #8310, #8218, #1942, #1852, #2599, #5072, #2113, #4253, #2866, #7044, #62, #708, #4895, #5598, #7746, #8617, #668, #755, #7134, #3513, #4390, #7086, #6336, #7219, #5023, #5685, #2067, #2248, #6469, #4342, #4210, #2201, #4296, #7880, #7835, #3556, #7796, #3600, #6378, #1500, #8442, #2777, #18, #1370, #2911, #6425, #104, #8531, #7178, #802, #3646, #2159, #9173, #4979, #2955, #9133 ) ),
 .UNSPECIFIED., .T., .F., .T. ) 
 B_SPLINE_SURFACE_WITH_KNOTS ( ( 4, 3, 4 ),
 ( 3, 2, 2, 2, 2, 2, 2, 2, 2, 2, 2, 2, 2, 2, 2, 2, 2, 2, 2, 2, 2, 2, 2, 2, 2, 2, 2, 2, 2, 2, 2, 2, 2, 2, 2, 2, 2, 2, 2, 2, 3 ),
 ( 0.000000000000000000, 0.5000000000000000000, 1.000000000000000000 ),
 ( 0.000000000000000000, 0.02500000000000000139, 0.05000000000000000278, 0.07499999999999999722, 0.1000000000000000056, 0.1250000000000000000, 0.1499999999999999944, 0.1749999999999999889, 0.2000000000000000111, 0.2250000000000000056, 0.2500000000000000000, 0.2750000000000000222, 0.2999999999999999889, 0.3250000000000000111, 0.3499999999999999778, 0.3750000000000000000, 0.4000000000000000222, 0.4249999999999999889, 0.4500000000000000111, 0.4749999999999999778, 0.5000000000000000000, 0.5250000000000000222, 0.5500000000000000444, 0.5749999999999999556, 0.5999999999999999778, 0.6250000000000000000, 0.6500000000000000222, 0.6750000000000000444, 0.6999999999999999556, 0.7249999999999999778, 0.7500000000000000000, 0.7750000000000000222, 0.8000000000000000444, 0.8249999999999999556, 0.8499999999999999778, 0.8750000000000000000, 0.9000000000000000222, 0.9250000000000000444, 0.9499999999999999556, 0.9749999999999999778, 1.000000000000000000 ),
 .UNSPECIFIED. ) 
 GEOMETRIC_REPRESENTATION_ITEM ( )  RATIONAL_B_SPLINE_SURFACE ( (
 ( 1.000000000000000000, 0.9238795325112867385, 1.000000000000000000, 0.9238795325112867385, 1.000000000000000000, 0.9238795325112867385, 1.000000000000000000, 0.9238795325112867385, 1.000000000000000000, 0.9238795325112867385, 1.000000000000000000, 0.9238795325112867385, 1.000000000000000000, 0.9238795325112867385, 1.000000000000000000, 0.9238795325112867385, 1.000000000000000000, 0.9238795325112867385, 1.000000000000000000, 0.9238795325112867385, 1.000000000000000000, 0.9238795325112867385, 1.000000000000000000, 0.9238795325112867385, 1.000000000000000000, 0.9238795325112867385, 1.000000000000000000, 0.9238795325112867385, 1.000000000000000000, 0.9238795325112867385, 1.000000000000000000, 0.9238795325112867385, 1.000000000000000000, 0.9238795325112867385, 1.000000000000000000, 0.9238795325112867385, 1.000000000000000000, 0.9238795325112867385, 1.000000000000000000, 0.9238795325112867385, 1.000000000000000000, 0.9238795325112867385, 1.000000000000000000, 0.9238795325112867385, 1.000000000000000000, 0.9238795325112867385, 1.000000000000000000, 0.9238795325112867385, 1.000000000000000000, 0.9238795325112867385, 1.000000000000000000, 0.9238795325112867385, 1.000000000000000000, 0.9238795325112867385, 1.000000000000000000, 0.9238795325112867385, 1.000000000000000000, 0.9238795325112867385, 1.000000000000000000, 0.9238795325112867385, 1.000000000000000000, 0.9238795325112867385, 1.000000000000000000, 0.9238795325112867385, 1.000000000000000000, 0.9238795325112867385, 1.000000000000000000, 0.9238795325112867385, 1.000000000000000000, 0.9238795325112867385, 1.000000000000000000, 0.9238795325112867385, 1.000000000000000000, 0.9238795325112867385, 1.000000000000000000, 0.9238795325112867385, 1.000000000000000000, 0.9238795325112867385, 1.000000000000000000, 0.9238795325112867385, 1.000000000000000000),
 ( 0.3333333333333333703, 0.3079598441704289313, 0.3333333333333333703, 0.3079598441704289313, 0.3333333333333333703, 0.3079598441704289313, 0.3333333333333333703, 0.3079598441704289313, 0.3333333333333333703, 0.3079598441704289313, 0.3333333333333333703, 0.3079598441704289313, 0.3333333333333333703, 0.3079598441704289313, 0.3333333333333333703, 0.3079598441704289313, 0.3333333333333333703, 0.3079598441704289313, 0.3333333333333333703, 0.3079598441704289313, 0.3333333333333333703, 0.3079598441704289313, 0.3333333333333333703, 0.3079598441704289313, 0.3333333333333333703, 0.3079598441704289313, 0.3333333333333333703, 0.3079598441704289313, 0.3333333333333333703, 0.3079598441704289313, 0.3333333333333333703, 0.3079598441704289313, 0.3333333333333333703, 0.3079598441704289313, 0.3333333333333333703, 0.3079598441704289313, 0.3333333333333333703, 0.3079598441704289313, 0.3333333333333333703, 0.3079598441704289313, 0.3333333333333333703, 0.3079598441704289313, 0.3333333333333333703, 0.3079598441704289313, 0.3333333333333333703, 0.3079598441704289313, 0.3333333333333333703, 0.3079598441704289313, 0.3333333333333333703, 0.3079598441704289313, 0.3333333333333333703, 0.3079598441704289313, 0.3333333333333333703, 0.3079598441704289313, 0.3333333333333333703, 0.3079598441704289313, 0.3333333333333333703, 0.3079598441704289313, 0.3333333333333333703, 0.3079598441704289313, 0.3333333333333333703, 0.3079598441704289313, 0.3333333333333333703, 0.3079598441704289313, 0.3333333333333333703, 0.3079598441704289313, 0.3333333333333333703, 0.3079598441704289313, 0.3333333333333333703, 0.3079598441704289313, 0.3333333333333333703, 0.3079598441704289313, 0.3333333333333333703, 0.3079598441704289313, 0.3333333333333333703, 0.3079598441704289313, 0.3333333333333333703, 0.3079598441704289313, 0.3333333333333333703, 0.3079598441704289313, 0.3333333333333333703),
 ( 0.3333333333333333703, 0.3079598441704289313, 0.3333333333333333703, 0.3079598441704289313, 0.3333333333333333703, 0.3079598441704289313, 0.3333333333333333703, 0.3079598441704289313, 0.3333333333333333703, 0.3079598441704289313, 0.3333333333333333703, 0.3079598441704289313, 0.3333333333333333703, 0.3079598441704289313, 0.3333333333333333703, 0.3079598441704289313, 0.3333333333333333703, 0.3079598441704289313, 0.3333333333333333703, 0.3079598441704289313, 0.3333333333333333703, 0.3079598441704289313, 0.3333333333333333703, 0.3079598441704289313, 0.3333333333333333703, 0.3079598441704289313, 0.3333333333333333703, 0.3079598441704289313, 0.3333333333333333703, 0.3079598441704289313, 0.3333333333333333703, 0.3079598441704289313, 0.3333333333333333703, 0.3079598441704289313, 0.3333333333333333703, 0.3079598441704289313, 0.3333333333333333703, 0.3079598441704289313, 0.3333333333333333703, 0.3079598441704289313, 0.3333333333333333703, 0.3079598441704289313, 0.3333333333333333703, 0.3079598441704289313, 0.3333333333333333703, 0.3079598441704289313, 0.3333333333333333703, 0.3079598441704289313, 0.3333333333333333703, 0.3079598441704289313, 0.3333333333333333703, 0.3079598441704289313, 0.3333333333333333703, 0.3079598441704289313, 0.3333333333333333703, 0.3079598441704289313, 0.3333333333333333703, 0.3079598441704289313, 0.3333333333333333703, 0.3079598441704289313, 0.3333333333333333703, 0.3079598441704289313, 0.3333333333333333703, 0.3079598441704289313, 0.3333333333333333703, 0.3079598441704289313, 0.3333333333333333703, 0.3079598441704289313, 0.3333333333333333703, 0.3079598441704289313, 0.3333333333333333703, 0.3079598441704289313, 0.3333333333333333703, 0.3079598441704289313, 0.3333333333333333703, 0.3079598441704289313, 0.3333333333333333703, 0.3079598441704289313, 0.3333333333333333703, 0.3079598441704289313, 0.3333333333333333703),
 ( 1.000000000000000000, 0.9238795325112867385, 1.000000000000000000, 0.9238795325112867385, 1.000000000000000000, 0.9238795325112867385, 1.000000000000000000, 0.9238795325112867385, 1.000000000000000000, 0.9238795325112867385, 1.000000000000000000, 0.9238795325112867385, 1.000000000000000000, 0.9238795325112867385, 1.000000000000000000, 0.9238795325112867385, 1.000000000000000000, 0.9238795325112867385, 1.000000000000000000, 0.9238795325112867385, 1.000000000000000000, 0.9238795325112867385, 1.000000000000000000, 0.9238795325112867385, 1.000000000000000000, 0.9238795325112867385, 1.000000000000000000, 0.9238795325112867385, 1.000000000000000000, 0.9238795325112867385, 1.000000000000000000, 0.9238795325112867385, 1.000000000000000000, 0.9238795325112867385, 1.000000000000000000, 0.9238795325112867385, 1.000000000000000000, 0.9238795325112867385, 1.000000000000000000, 0.9238795325112867385, 1.000000000000000000, 0.9238795325112867385, 1.000000000000000000, 0.9238795325112867385, 1.000000000000000000, 0.9238795325112867385, 1.000000000000000000, 0.9238795325112867385, 1.000000000000000000, 0.9238795325112867385, 1.000000000000000000, 0.9238795325112867385, 1.000000000000000000, 0.9238795325112867385, 1.000000000000000000, 0.9238795325112867385, 1.000000000000000000, 0.9238795325112867385, 1.000000000000000000, 0.9238795325112867385, 1.000000000000000000, 0.9238795325112867385, 1.000000000000000000, 0.9238795325112867385, 1.000000000000000000, 0.9238795325112867385, 1.000000000000000000, 0.9238795325112867385, 1.000000000000000000, 0.9238795325112867385, 1.000000000000000000, 0.9238795325112867385, 1.000000000000000000, 0.9238795325112867385, 1.000000000000000000, 0.9238795325112867385, 1.000000000000000000, 0.9238795325112867385, 1.000000000000000000, 0.9238795325112867385, 1.000000000000000000),
 ( 0.3333333333333333703, 0.3079598441704289313, 0.3333333333333333703, 0.3079598441704289313, 0.3333333333333333703, 0.3079598441704289313, 0.3333333333333333703, 0.3079598441704289313, 0.3333333333333333703, 0.3079598441704289313, 0.3333333333333333703, 0.3079598441704289313, 0.3333333333333333703, 0.3079598441704289313, 0.3333333333333333703, 0.3079598441704289313, 0.3333333333333333703, 0.3079598441704289313, 0.3333333333333333703, 0.3079598441704289313, 0.3333333333333333703, 0.3079598441704289313, 0.3333333333333333703, 0.3079598441704289313, 0.3333333333333333703, 0.3079598441704289313, 0.3333333333333333703, 0.3079598441704289313, 0.3333333333333333703, 0.3079598441704289313, 0.3333333333333333703, 0.3079598441704289313, 0.3333333333333333703, 0.3079598441704289313, 0.3333333333333333703, 0.3079598441704289313, 0.3333333333333333703, 0.3079598441704289313, 0.3333333333333333703, 0.3079598441704289313, 0.3333333333333333703, 0.3079598441704289313, 0.3333333333333333703, 0.3079598441704289313, 0.3333333333333333703, 0.3079598441704289313, 0.3333333333333333703, 0.3079598441704289313, 0.3333333333333333703, 0.3079598441704289313, 0.3333333333333333703, 0.3079598441704289313, 0.3333333333333333703, 0.3079598441704289313, 0.3333333333333333703, 0.3079598441704289313, 0.3333333333333333703, 0.3079598441704289313, 0.3333333333333333703, 0.3079598441704289313, 0.3333333333333333703, 0.3079598441704289313, 0.3333333333333333703, 0.3079598441704289313, 0.3333333333333333703, 0.3079598441704289313, 0.3333333333333333703, 0.3079598441704289313, 0.3333333333333333703, 0.3079598441704289313, 0.3333333333333333703, 0.3079598441704289313, 0.3333333333333333703, 0.3079598441704289313, 0.3333333333333333703, 0.3079598441704289313, 0.3333333333333333703, 0.3079598441704289313, 0.3333333333333333703, 0.3079598441704289313, 0.3333333333333333703),
 ( 0.3333333333333333703, 0.3079598441704289313, 0.3333333333333333703, 0.3079598441704289313, 0.3333333333333333703, 0.3079598441704289313, 0.3333333333333333703, 0.3079598441704289313, 0.3333333333333333703, 0.3079598441704289313, 0.3333333333333333703, 0.3079598441704289313, 0.3333333333333333703, 0.3079598441704289313, 0.3333333333333333703, 0.3079598441704289313, 0.3333333333333333703, 0.3079598441704289313, 0.3333333333333333703, 0.3079598441704289313, 0.3333333333333333703, 0.3079598441704289313, 0.3333333333333333703, 0.3079598441704289313, 0.3333333333333333703, 0.3079598441704289313, 0.3333333333333333703, 0.3079598441704289313, 0.3333333333333333703, 0.3079598441704289313, 0.3333333333333333703, 0.3079598441704289313, 0.3333333333333333703, 0.3079598441704289313, 0.3333333333333333703, 0.3079598441704289313, 0.3333333333333333703, 0.3079598441704289313, 0.3333333333333333703, 0.3079598441704289313, 0.3333333333333333703, 0.3079598441704289313, 0.3333333333333333703, 0.3079598441704289313, 0.3333333333333333703, 0.3079598441704289313, 0.3333333333333333703, 0.3079598441704289313, 0.3333333333333333703, 0.3079598441704289313, 0.3333333333333333703, 0.3079598441704289313, 0.3333333333333333703, 0.3079598441704289313, 0.3333333333333333703, 0.3079598441704289313, 0.3333333333333333703, 0.3079598441704289313, 0.3333333333333333703, 0.3079598441704289313, 0.3333333333333333703, 0.3079598441704289313, 0.3333333333333333703, 0.3079598441704289313, 0.3333333333333333703, 0.3079598441704289313, 0.3333333333333333703, 0.3079598441704289313, 0.3333333333333333703, 0.3079598441704289313, 0.3333333333333333703, 0.3079598441704289313, 0.3333333333333333703, 0.3079598441704289313, 0.3333333333333333703, 0.3079598441704289313, 0.3333333333333333703, 0.3079598441704289313, 0.3333333333333333703, 0.3079598441704289313, 0.3333333333333333703),
 ( 1.000000000000000000, 0.9238795325112867385, 1.000000000000000000, 0.9238795325112867385, 1.000000000000000000, 0.9238795325112867385, 1.000000000000000000, 0.9238795325112867385, 1.000000000000000000, 0.9238795325112867385, 1.000000000000000000, 0.9238795325112867385, 1.000000000000000000, 0.9238795325112867385, 1.000000000000000000, 0.9238795325112867385, 1.000000000000000000, 0.9238795325112867385, 1.000000000000000000, 0.9238795325112867385, 1.000000000000000000, 0.9238795325112867385, 1.000000000000000000, 0.9238795325112867385, 1.000000000000000000, 0.9238795325112867385, 1.000000000000000000, 0.9238795325112867385, 1.000000000000000000, 0.9238795325112867385, 1.000000000000000000, 0.9238795325112867385, 1.000000000000000000, 0.9238795325112867385, 1.000000000000000000, 0.9238795325112867385, 1.000000000000000000, 0.9238795325112867385, 1.000000000000000000, 0.9238795325112867385, 1.000000000000000000, 0.9238795325112867385, 1.000000000000000000, 0.9238795325112867385, 1.000000000000000000, 0.9238795325112867385, 1.000000000000000000, 0.9238795325112867385, 1.000000000000000000, 0.9238795325112867385, 1.000000000000000000, 0.9238795325112867385, 1.000000000000000000, 0.9238795325112867385, 1.000000000000000000, 0.9238795325112867385, 1.000000000000000000, 0.9238795325112867385, 1.000000000000000000, 0.9238795325112867385, 1.000000000000000000, 0.9238795325112867385, 1.000000000000000000, 0.9238795325112867385, 1.000000000000000000, 0.9238795325112867385, 1.000000000000000000, 0.9238795325112867385, 1.000000000000000000, 0.9238795325112867385, 1.000000000000000000, 0.9238795325112867385, 1.000000000000000000, 0.9238795325112867385, 1.000000000000000000, 0.9238795325112867385, 1.000000000000000000, 0.9238795325112867385, 1.000000000000000000, 0.9238795325112867385, 1.000000000000000000) ) ) 
 REPRESENTATION_ITEM ( '' )  SURFACE ( )  );
#2954=CARTESIAN_POINT ( 'NONE',  ( 0.01814118441321408565, -6.249340926099360871, -3.500000000000000000 ) ) ;
#2955=CARTESIAN_POINT ( 'NONE',  ( -3.492485675378536047, -8.149340926099361226, -1.467888652719048670 ) ) ;
#2963=CARTESIAN_POINT ( 'NONE',  ( -4.000000000000000000, -0.2493409260993606769, -0.01814118441321865144 ) ) ;
#2971=CARTESIAN_POINT ( 'NONE',  ( -0.01814118441321365544, -2.249340926099361315, 3.500000000000000000 ) ) ;
#2973=CARTESIAN_POINT ( 'NONE',  ( -1.224499502706077880, -1.549340926099361804, -3.007514324621463064 ) ) ;
#2975=DIRECTION ( 'NONE',  ( 0.000000000000000000, -0.9973637043974449279, -0.07256473765270717025 ) ) ;
#2976=CARTESIAN_POINT ( 'NONE',  ( -4.007514324621467949, -1.949340926099360827, 1.638713065079161924 ) ) ;
#2989=CARTESIAN_POINT ( 'NONE',  ( 2.108492589042352705, -3.950659073900640195, -2.134148098076933397 ) ) ;
#2999=CARTESIAN_POINT ( 'NONE',  ( 3.500000000000000000, -5.849340926099361404, 0.01814118441321387054 ) ) ;
#3011=CARTESIAN_POINT ( 'NONE',  ( -0.01814118441313417734, -7.350659073900637885, -4.000000000000000000 ) ) ;
#3021=CARTESIAN_POINT ( 'NONE',  ( 2.134148098076933397, -1.950659073900639306, 2.108492589042352261 ) ) ;
#3022=UNCERTAINTY_MEASURE_WITH_UNIT (LENGTH_MEASURE( 1.000000000000000082E-05 ), #2152, 'distance_accuracy_value', 'NONE');
#3024=CARTESIAN_POINT ( 'NONE',  ( -4.000000000000000000, -0.2493409260993606769, -0.01814118441321865144 ) ) ;
#3029=CARTESIAN_POINT ( 'NONE',  ( -3.500000000000000000, -3.449340926099361049, -0.01814118441321344033 ) ) ;
#3035=CARTESIAN_POINT ( 'NONE',  ( 0.01814118441321938349, -6.249340926099361759, -4.000000000000000000 ) ) ;
#3040=CARTESIAN_POINT ( 'NONE',  ( 1.260781871532430598, -6.650659073900641260, 2.992485675378564469 ) ) ;
#3048=CARTESIAN_POINT ( 'NONE',  ( -3.507514324621464397, -3.549340926099361582, 1.431606283892619347 ) ) ;
#3052=CARTESIAN_POINT ( 'NONE',  ( -2.462045979635576920, -6.449340926099361937, -2.487701488670255756 ) ) ;
#3061=CARTESIAN_POINT ( 'NONE',  ( -0.01814118441313417734, -4.150659073900638596, -4.000000000000000000 ) ) ;
#3071=CARTESIAN_POINT ( 'NONE',  ( -1.260781871532431708, -1.050659073900639617, -2.992485675378564469 ) ) ;
#3072=CARTESIAN_POINT ( 'NONE',  ( -1.638713065079163034, -1.549340926099360916, -4.007514324621466173 ) ) ;
#3075=CARTESIAN_POINT ( 'NONE',  ( -1.431606283892620235, -3.149340926099361671, -3.507514324621463953 ) ) ;
#3079=CARTESIAN_POINT ( 'NONE',  ( 4.000000000000000000, -4.249340926099360871, 0.01814118441321914063 ) ) ;
#3083=CARTESIAN_POINT ( 'NONE',  ( 2.108492589042352705, -7.150659073900638596, -2.134148098076933397 ) ) ;
#3090=CARTESIAN_POINT ( 'NONE',  ( 0.01814118441321408565, -3.049340926099361138, -3.500000000000000000 ) ) ;
#3102=CARTESIAN_POINT ( 'NONE',  ( 1.674995433905515085, -5.050659073900638951, 3.992485675378568022 ) ) ;
#3115=CARTESIAN_POINT ( 'NONE',  ( 3.007514324621436863, -5.250659073900640017, 1.224499502706140719 ) ) ;
#3118=CARTESIAN_POINT ( 'NONE',  ( -3.250000000000000444, 0.000000000000000000, -3.404030812060692501E-14 ) ) ;
#3120=CARTESIAN_POINT ( 'NONE',  ( 1.467888652719048226, -4.549340926099360694, -3.492485675378535603 ) ) ;
#3125=CARTESIAN_POINT ( 'NONE',  ( 1.638713065079161924, -7.149340926099361226, 4.007514324621467949 ) ) ;
#3130=CARTESIAN_POINT ( 'NONE',  ( 2.108492589042352705, -5.550659073900639839, -2.134148098076933397 ) ) ;
#3142=CARTESIAN_POINT ( 'NONE',  ( 3.507514324621465285, -1.149340926099361226, -1.431606283892619125 ) ) ;
#3153=CARTESIAN_POINT ( 'NONE',  ( 2.841254879263473310, -3.550659073900638063, 2.815599370228907272 ) ) ;
#3161=CARTESIAN_POINT ( 'NONE',  ( 0.01814118441314514080, -3.350659073900639662, 3.000000000000000444 ) ) ;
#3165=LINE ( 'NONE', #7990, #1845 ) ;
#3166=CARTESIAN_POINT ( 'NONE',  ( 1.431606283892619347, -3.949340926099361049, 3.507514324621464397 ) ) ;
#3171=CARTESIAN_POINT ( 'NONE',  ( 2.841254879263533262, -2.849340926099360960, -2.815599370228847320 ) ) ;
#3175=CARTESIAN_POINT ( 'NONE',  ( 3.500000000000000000, -5.350659073900638774, -0.01814118441313969030 ) ) ;
#3185=CARTESIAN_POINT ( 'NONE',  ( 2.462045979635577364, -5.649340926099361226, 2.487701488670255312 ) ) ;
#3186=DIRECTION ( 'NONE',  ( 0.000000000000000000, 0.9973637043974448169, 0.07256473765270714249 ) ) ;
#3196=CARTESIAN_POINT ( 'NONE',  ( 1.674995433905601239, -1.349340926099360960, -3.992485675378532939 ) ) ;
#3207=CARTESIAN_POINT ( 'NONE',  ( -2.992485675378564469, 0.1493409260993606713, 1.260781871532430820 ) ) ;
#3211=CARTESIAN_POINT ( 'NONE',  ( -2.487701488670255312, -0.4493409260993610488, 2.462045979635577808 ) ) ;
#3215=CARTESIAN_POINT ( 'NONE',  ( -4.000000000000000000, -3.449340926099361049, -0.01814118441321865144 ) ) ;
#3219=CARTESIAN_POINT ( 'NONE',  ( 1.467888652718972731, -1.850659073900638996, 3.492485675378566246 ) ) ;
#3229=CARTESIAN_POINT ( 'NONE',  ( -2.134148098076978251, -2.049340926099361138, 2.108492589042307408 ) ) ;
#3242=CARTESIAN_POINT ( 'NONE',  ( 1.638713065079161924, -0.7493409260993607601, 4.007514324621467949 ) ) ;
#3250=CARTESIAN_POINT ( 'NONE',  ( 2.108492589042352705, -5.550659073900639839, -2.134148098076933397 ) ) ;
#3259=CARTESIAN_POINT ( 'NONE',  ( -2.487701488670255312, -5.249340926099360871, 2.462045979635577808 ) ) ;
#3262=CARTESIAN_POINT ( 'NONE',  ( -0.01814118441313947866, -7.350659073900638774, -3.500000000000000000 ) ) ;
#3266=CARTESIAN_POINT ( 'NONE',  ( 3.500000000000000000, -3.750659073900639129, -0.01814118441313969030 ) ) ;
#3273=CARTESIAN_POINT ( 'NONE',  ( -3.000000000000000444, -0.2493409260993614540, -0.01814118441320822922 ) ) ;
#3290=CARTESIAN_POINT ( 'NONE',  ( 0.01814118441321938349, -6.249340926099361759, -4.000000000000000000 ) ) ;
#3299=CARTESIAN_POINT ( 'NONE',  ( -2.108492589042352261, -6.350659073900638774, 2.134148098076933397 ) ) ;
#3307=CARTESIAN_POINT ( 'NONE',  ( -3.492485675378536047, -6.549340926099363358, -1.467888652719048670 ) ) ;
#3311=CARTESIAN_POINT ( 'NONE',  ( -1.431606283892693066, -1.650659073900638818, 3.507514324621434199 ) ) ;
#3316=EDGE_CURVE ( 'NONE', #845, #183, #5503, .T. ) ;
#3323=CARTESIAN_POINT ( 'NONE',  ( 0.01814118441320878086, -4.649340926099361226, -3.000000000000000444 ) ) ;
#3327=CARTESIAN_POINT ( 'NONE',  ( -1.925759277493323207, -9.035843541029837430E-14, 2.922632427747480222 ) ) ;
#3339=CARTESIAN_POINT ( 'NONE',  ( -2.462045979635576920, -3.249340926099361315, -2.487701488670255756 ) ) ;
#3340=CARTESIAN_POINT ( 'NONE',  ( 3.992485675378533383, -7.349340926099363180, 1.674995433905599462 ) ) ;
#3347=CARTESIAN_POINT ( 'NONE',  ( 2.487701488670203354, -3.550659073900638951, 2.462045979635629323 ) ) ;
#3352=CARTESIAN_POINT ( 'NONE',  ( 3.492485675378535603, -7.349340926099362292, 1.467888652719046672 ) ) ;
#3357=CARTESIAN_POINT ( 'NONE',  ( -2.462045979635576920, -6.449340926099361937, -2.487701488670255756 ) ) ;
#3360=CARTESIAN_POINT ( 'NONE',  ( -1.431606283892693066, -4.850659073900638774, 3.507514324621434199 ) ) ;
#3364=CARTESIAN_POINT ( 'NONE',  ( 3.492485675378566690, -5.450659073900639306, -1.467888652718972287 ) ) ;
#3368=CARTESIAN_POINT ( 'NONE',  ( -3.500000000000000000, -8.249340926099360871, -0.01814118441321344033 ) ) ;
#3380=CARTESIAN_POINT ( 'NONE',  ( 1.467888652719048226, -6.149340926099360338, -3.492485675378536047 ) ) ;
#3381=CARTESIAN_POINT ( 'NONE',  ( -2.841254879263533262, -5.249340926099361759, 2.815599370228847764 ) ) ;
#3388=( GEOMETRIC_REPRESENTATION_CONTEXT ( 3 ) GLOBAL_UNCERTAINTY_ASSIGNED_CONTEXT ( ( #8034 ) ) GLOBAL_UNIT_ASSIGNED_CONTEXT ( ( #8657, #2288, #11 ) ) REPRESENTATION_CONTEXT ( 'NONE', 'WORKASPACE' ) );
#3392=CARTESIAN_POINT ( 'NONE',  ( 1.224499502706142273, -7.250659073900640905, -3.007514324621435531 ) ) ;
#3397=CARTESIAN_POINT ( 'NONE',  ( -2.487701488670255312, -6.849340926099361404, 2.462045979635577808 ) ) ;
#3401=CARTESIAN_POINT ( 'NONE',  ( 1.638713065079247855, -4.050659073900639839, -4.007514324621431534 ) ) ;
#3403=CARTESIAN_POINT ( 'NONE',  ( -2.487701488670255312, -3.649340926099361226, 2.462045979635577808 ) ) ;
#3406=CARTESIAN_POINT ( 'NONE',  ( -4.000000000000000000, -4.550659073900638951, 0.01814118441313491634 ) ) ;
#3413=CARTESIAN_POINT ( 'NONE',  ( 2.108492589042352705, -2.350659073900639218, -2.134148098076933397 ) ) ;
#3427=CARTESIAN_POINT ( 'NONE',  ( 3.507514324621465285, -1.149340926099361226, -1.431606283892619125 ) ) ;
#3428=CARTESIAN_POINT ( 'NONE',  ( 2.815599370228847320, -5.649340926099361226, 2.841254879263533262 ) ) ;
#3436=CARTESIAN_POINT ( 'NONE',  ( -2.841254879263473310, -1.150659073900638374, -2.815599370228907716 ) ) ;
#3445=CARTESIAN_POINT ( 'NONE',  ( -3.500000000000000000, -6.649340926099361226, -0.01814118441321344033 ) ) ;
#3449=CARTESIAN_POINT ( 'NONE',  ( 4.000000000000000000, -2.150659073900639040, -0.01814118441313441674 ) ) ;
#3455=CARTESIAN_POINT ( 'NONE',  ( -3.000000000000000444, -6.649340926099362115, -0.01814118441320822922 ) ) ;
#3464=CARTESIAN_POINT ( 'NONE',  ( -1.467888652719046449, -0.5493409260993611376, 3.492485675378536047 ) ) ;
#3467=CARTESIAN_POINT ( 'NONE',  ( -0.01814118441321365544, -0.6493409260993610044, 3.500000000000000000 ) ) ;
#3468=CARTESIAN_POINT ( 'NONE',  ( -1.674995433905599462, -6.949340926099362825, 3.992485675378533383 ) ) ;
#3477=CARTESIAN_POINT ( 'NONE',  ( -2.487701488670202910, -4.350659073900638774, -2.462045979635629767 ) ) ;
#3488=CARTESIAN_POINT ( 'NONE',  ( 1.260781871532495657, -6.149340926099362115, -2.992485675378538268 ) ) ;
#3491=CARTESIAN_POINT ( 'NONE',  ( 0.01814118441313467001, -3.350659073900638774, 4.000000000000000000 ) ) ;
#3494=CARTESIAN_POINT ( 'NONE',  ( -3.500000000000000000, -8.000000000000000000, -3.665958595716611867E-14 ) ) ;
#3500=CARTESIAN_POINT ( 'NONE',  ( -1.224499502706077880, -7.949340926099362825, -3.007514324621463064 ) ) ;
#3512=CARTESIAN_POINT ( 'NONE',  ( -2.462045979635576920, -1.649340926099361004, -2.487701488670255756 ) ) ;
#3513=CARTESIAN_POINT ( 'NONE',  ( 0.01814118441321408565, -4.649340926099361226, -3.500000000000000000 ) ) ;
#3519=CARTESIAN_POINT ( 'NONE',  ( -2.487701488670202910, -5.950659073900639306, -2.462045979635629767 ) ) ;
#3526=EDGE_CURVE ( 'NONE', #2600, #3793, #1951, .T. ) ;
#3531=CARTESIAN_POINT ( 'NONE',  ( -2.992485675378538268, -6.549340926099361582, -1.260781871532495879 ) ) ;
#3534=CARTESIAN_POINT ( 'NONE',  ( 1.674995433905515085, -0.2506590739006385182, 3.992485675378568022 ) ) ;
#3541=CARTESIAN_POINT ( 'NONE',  ( 1.224499502706077214, -7.149340926099361226, 3.007514324621463508 ) ) ;
#3554=CARTESIAN_POINT ( 'NONE',  ( -2.074671974031725874, -3.217773792136106728E-17, 2.904849880052185362 ) ) ;
#3556=CARTESIAN_POINT ( 'NONE',  ( 0.01814118441321408565, -6.249340926099360871, -3.500000000000000000 ) ) ;
#3565=CARTESIAN_POINT ( 'NONE',  ( 2.462045979635629767, -5.550659073900639839, -2.487701488670203354 ) ) ;
#3576=CARTESIAN_POINT ( 'NONE',  ( 2.108492589042307408, -2.449340926099361937, 2.134148098076978251 ) ) ;
#3579=CARTESIAN_POINT ( 'NONE',  ( 3.992485675378568910, -2.250659073900638685, -1.674995433905514863 ) ) ;
#3587=CARTESIAN_POINT ( 'NONE',  ( -0.01814118441314477650, -0.9506590739006395285, -3.000000000000000444 ) ) ;
#3597=CARTESIAN_POINT ( 'NONE',  ( -3.750000000000003109, -1.355252715626601757E-17, 0.3087531627310677318 ) ) ;
#3600=CARTESIAN_POINT ( 'NONE',  ( -2.462045979635576920, -6.449340926099361937, -2.487701488670255756 ) ) ;
#3608=CARTESIAN_POINT ( 'NONE',  ( 1.638713065079247855, -0.8506590739006385515, -4.007514324621431534 ) ) ;
#3622=CARTESIAN_POINT ( 'NONE',  ( 1.260781871532495657, -4.549340926099363358, -2.992485675378538268 ) ) ;
#3623=CARTESIAN_POINT ( 'NONE',  ( -3.500000000000000000, -8.000000000000000000, -3.665958595716611867E-14 ) ) ;
#3626=CARTESIAN_POINT ( 'NONE',  ( -4.000000000000000000, -7.750659073900639129, 0.01814118441313491634 ) ) ;
#3634=CARTESIAN_POINT ( 'NONE',  ( 2.462045979635629767, -0.7506590739006389068, -2.487701488670203354 ) ) ;
#3645=CARTESIAN_POINT ( 'NONE',  ( 1.431606283892619125, -7.149340926099362115, 3.507514324621464397 ) ) ;
#3646=CARTESIAN_POINT ( 'NONE',  ( 1.467888652719048226, -7.749340926099361759, -3.492485675378536047 ) ) ;
#3654=CARTESIAN_POINT ( 'NONE',  ( -4.007514324621431534, -7.650659073900639484, -1.638713065079248521 ) ) ;
#3658=EDGE_CURVE ( 'NONE', #7146, #3793, #531, .T. ) ;
#3662=CARTESIAN_POINT ( 'NONE',  ( 2.462045979635577364, -0.8493409260993610710, 2.487701488670255312 ) ) ;
#3664=CARTESIAN_POINT ( 'NONE',  ( -2.992485675378538268, -1.749340926099361981, -1.260781871532495879 ) ) ;
#3668=CARTESIAN_POINT ( 'NONE',  ( -2.841254879263533262, -2.049340926099361138, 2.815599370228847764 ) ) ;
#3679=CARTESIAN_POINT ( 'NONE',  ( -1.224499502706140497, -6.450659073900641971, 3.007514324621436863 ) ) ;
#3687=CARTESIAN_POINT ( 'NONE',  ( 3.507514324621465285, -4.349340926099361404, -1.431606283892619125 ) ) ;
#3690=CARTESIAN_POINT ( 'NONE',  ( -1.431606283892620235, -6.349340926099360516, -3.507514324621463953 ) ) ;
#3702=CARTESIAN_POINT ( 'NONE',  ( 1.638713065079161924, -0.7493409260993607601, 4.007514324621467949 ) ) ;
#3711=CARTESIAN_POINT ( 'NONE',  ( 1.467888652719048226, -1.349340926099361182, -3.492485675378536047 ) ) ;
#3713=CARTESIAN_POINT ( 'NONE',  ( 0.01814118441314514080, -4.950659073900641083, 3.000000000000000444 ) ) ;
#3716=CARTESIAN_POINT ( 'NONE',  ( -4.000000000000000000, -1.849340926099360738, -0.01814118441321865144 ) ) ;
#3720=CARTESIAN_POINT ( 'NONE',  ( 3.492485675378535603, -4.149340926099362115, 1.467888652719046672 ) ) ;
#3727=CARTESIAN_POINT ( 'NONE',  ( -2.815599370228846876, -3.249340926099360871, -2.841254879263533262 ) ) ;
#3731=CARTESIAN_POINT ( 'NONE',  ( -3.492485675378566246, 0.1493409260993610876, 1.467888652718973397 ) ) ;
#3735=APPLICATION_CONTEXT ( 'automotive_design' ) ;
#3742=CARTESIAN_POINT ( 'NONE',  ( -2.487701488670255312, -6.849340926099361404, 2.462045979635577808 ) ) ;
#3745=CARTESIAN_POINT ( 'NONE',  ( 1.467888652719048226, -7.749340926099361759, -3.492485675378536047 ) ) ;
#3753=CARTESIAN_POINT ( 'NONE',  ( -2.815599370228907272, -6.350659073900638774, 2.841254879263473754 ) ) ;
#3760=CARTESIAN_POINT ( 'NONE',  ( -0.01814118441321365544, -0.6493409260993610044, 3.500000000000000000 ) ) ;
#3762=CARTESIAN_POINT ( 'NONE',  ( 1.260781871532430598, -0.2506590739006394064, 2.992485675378564469 ) ) ;
#3765=CARTESIAN_POINT ( 'NONE',  ( 1.638713065079247855, -7.250659073900640017, -4.007514324621431534 ) ) ;
#3770=CARTESIAN_POINT ( 'NONE',  ( 2.462045979635577364, -4.049340926099360694, 2.487701488670255312 ) ) ;
#3774=CARTESIAN_POINT ( 'NONE',  ( 1.674995433905601239, -4.549340926099363358, -3.992485675378532939 ) ) ;
#3779=CARTESIAN_POINT ( 'NONE',  ( 3.500000000000000000, -0.5506590739006389512, -0.01814118441313969030 ) ) ;
#3788=CARTESIAN_POINT ( 'NONE',  ( -1.431606283892620235, -4.749340926099363536, -3.507514324621463953 ) ) ;
#3793=VERTEX_POINT ( 'NONE', #7758 ) ;
#3801=CARTESIAN_POINT ( 'NONE',  ( 1.638713065079247855, -5.650659073900638596, -4.007514324621431534 ) ) ;
#3808=CARTESIAN_POINT ( 'NONE',  ( -1.260781871532431708, -2.650659073900639928, -2.992485675378564469 ) ) ;
#3813=CARTESIAN_POINT ( 'NONE',  ( -3.492485675378535603, -4.949340926099361049, -1.467888652719048670 ) ) ;
#3818=CARTESIAN_POINT ( 'NONE',  ( 0.01814118441321938349, -4.649340926099361226, -4.000000000000000000 ) ) ;
#3822=CARTESIAN_POINT ( 'NONE',  ( -1.467888652718973619, -1.050659073900638951, -3.492485675378565801 ) ) ;
#3825=CARTESIAN_POINT ( 'NONE',  ( -3.500000000000000000, -2.950659073900639306, 0.01814118441314012051 ) ) ;
#3826=STYLED_ITEM ( 'NONE', ( #7037 ), #542 ) ;
#3829=CARTESIAN_POINT ( 'NONE',  ( 2.487701488670255756, -1.249340926099361093, -2.462045979635577364 ) ) ;
#3842=CARTESIAN_POINT ( 'NONE',  ( 4.000000000000000000, -5.350659073900637885, -0.01814118441313441674 ) ) ;
#3856=CARTESIAN_POINT ( 'NONE',  ( 1.260781871532430598, -1.850659073900639884, 2.992485675378564469 ) ) ;
#3860=CARTESIAN_POINT ( 'NONE',  ( 3.507514324621465285, -2.749340926099361315, -1.431606283892619347 ) ) ;
#3865=CARTESIAN_POINT ( 'NONE',  ( 2.815599370228847320, -5.649340926099361226, 2.841254879263533262 ) ) ;
#3871=CARTESIAN_POINT ( 'NONE',  ( -0.01814118441313947866, -5.750659073900639129, -3.500000000000000000 ) ) ;
#3875=CARTESIAN_POINT ( 'NONE',  ( -0.01814118441313947866, -0.9506590739006390844, -3.500000000000000000 ) ) ;
#3881=CARTESIAN_POINT ( 'NONE',  ( -1.467888652719046449, -5.349340926099361404, 3.492485675378536047 ) ) ;
#3893=CARTESIAN_POINT ( 'NONE',  ( 4.007514324621469726, -1.149340926099360782, -1.638713065079161257 ) ) ;
#3902=CARTESIAN_POINT ( 'NONE',  ( 3.000000000000000444, -2.150659073900639484, -0.01814118441314496039 ) ) ;
#3907=CARTESIAN_POINT ( 'NONE',  ( 2.462045979635577364, -5.649340926099361226, 2.487701488670255312 ) ) ;
#3911=CARTESIAN_POINT ( 'NONE',  ( -3.992485675378532939, -3.349340926099360960, -1.674995433905601683 ) ) ;
#3916=CARTESIAN_POINT ( 'NONE',  ( 3.492485675378566690, -5.450659073900639306, -1.467888652718972287 ) ) ;
#3920=CARTESIAN_POINT ( 'NONE',  ( 3.492485675378566690, -2.250659073900639573, -1.467888652718972287 ) ) ;
#3926=CARTESIAN_POINT ( 'NONE',  ( 2.134148098076978251, -1.249340926099361537, -2.108492589042307408 ) ) ;
#3932=CARTESIAN_POINT ( 'NONE',  ( -1.953518037137212504, -4.474939649319626956E-16, 2.844108989334067861 ) ) ;
#3940=CARTESIAN_POINT ( 'NONE',  ( 3.992485675378533383, -4.149340926099362115, 1.674995433905599462 ) ) ;
#3948=CARTESIAN_POINT ( 'NONE',  ( 1.260781871532430598, -6.650659073900641260, 2.992485675378564469 ) ) ;
#3953=CARTESIAN_POINT ( 'NONE',  ( -1.431606283892620235, -6.349340926099361404, -3.507514324621463953 ) ) ;
#3958=CARTESIAN_POINT ( 'NONE',  ( -3.492485675378536047, -3.349340926099361404, -1.467888652719048670 ) ) ;
#3962=CARTESIAN_POINT ( 'NONE',  ( 2.487701488670203354, -5.150659073900639484, 2.462045979635629323 ) ) ;
#3972=CARTESIAN_POINT ( 'NONE',  ( -2.992485675378538268, -3.349340926099362292, -1.260781871532495879 ) ) ;
#3988=CARTESIAN_POINT ( 'NONE',  ( 3.492485675378536047, -0.9493409260993610488, 1.467888652719046672 ) ) ;
#3995=CARTESIAN_POINT ( 'NONE',  ( -0.01814118441314477650, -5.750659073900639129, -3.000000000000000444 ) ) ;
#4005=CARTESIAN_POINT ( 'NONE',  ( -0.01814118441321365544, -5.449340926099361937, 3.500000000000000000 ) ) ;
#4008=CARTESIAN_POINT ( 'NONE',  ( 2.462045979635629767, -7.150659073900639484, -2.487701488670203354 ) ) ;
#4013=CARTESIAN_POINT ( 'NONE',  ( -3.507514324621433754, -1.250659073900639129, -1.431606283892695064 ) ) ;
#4019=CARTESIAN_POINT ( 'NONE',  ( -2.134148098076978251, -3.649340926099361671, 2.108492589042307408 ) ) ;
#4024=CARTESIAN_POINT ( 'NONE',  ( -2.122541484417015401, -1.321938709600337619E-17, 2.648722836990621499 ) ) ;
#4026=CARTESIAN_POINT ( 'NONE',  ( 0.000000000000000000, 0.000000000000000000, 0.000000000000000000 ) ) ;
#4032=DIRECTION ( 'NONE',  ( -1.044949058366720058E-14, -0.07256473765270715637, 0.9973637043974449279 ) ) ;
#4034=CARTESIAN_POINT ( 'NONE',  ( 1.467888652719048226, -4.549340926099360694, -3.492485675378536047 ) ) ;
#4035=CARTESIAN_POINT ( 'NONE',  ( 2.841254879263533262, -6.049340926099361582, -2.815599370228847320 ) ) ;
#4044=CARTESIAN_POINT ( 'NONE',  ( -1.431606283892693066, -3.250659073900639129, 3.507514324621434199 ) ) ;
#4052=CARTESIAN_POINT ( 'NONE',  ( -1.431606283892620235, -4.749340926099363536, -3.507514324621463953 ) ) ;
#4055=CARTESIAN_POINT ( 'NONE',  ( -1.467888652718973619, -5.850659073900639662, -3.492485675378565801 ) ) ;
#4059=CARTESIAN_POINT ( 'NONE',  ( 1.467888652718972731, -5.050659073900638951, 3.492485675378566246 ) ) ;
#4064=CARTESIAN_POINT ( 'NONE',  ( 3.000000000000000444, -4.249340926099360871, 0.01814118441320859698 ) ) ;
#4079=CARTESIAN_POINT ( 'NONE',  ( 3.500000000000000000, -5.849340926099361404, 0.01814118441321387054 ) ) ;
#4080=CARTESIAN_POINT ( 'NONE',  ( -0.01814118441321365544, -0.6493409260993610044, 3.500000000000000000 ) ) ;
#4088=CARTESIAN_POINT ( 'NONE',  ( 0.01814118441314514080, -6.550659073900640728, 3.000000000000000444 ) ) ;
#4092=CARTESIAN_POINT ( 'NONE',  ( -2.462045979635576920, -6.449340926099361937, -2.487701488670255756 ) ) ;
#4098=CARTESIAN_POINT ( 'NONE',  ( -3.507514324621464397, -5.149340926099360338, 1.431606283892619347 ) ) ;
#4102=CARTESIAN_POINT ( 'NONE',  ( 1.638713065079247855, -5.650659073900638596, -4.007514324621431534 ) ) ;
#4108=CARTESIAN_POINT ( 'NONE',  ( -1.224499502706077880, -4.749340926099361759, -3.007514324621463064 ) ) ;
#4119=CARTESIAN_POINT ( 'NONE',  ( -2.487701488670255312, -2.049340926099361582, 2.462045979635577808 ) ) ;
#4120=CARTESIAN_POINT ( 'NONE',  ( 2.462045979635577364, -2.449340926099361049, 2.487701488670255312 ) ) ;
#4128=CARTESIAN_POINT ( 'NONE',  ( 1.224499502706142273, -5.650659073900639484, -3.007514324621435531 ) ) ;
#4134=CARTESIAN_POINT ( 'NONE',  ( 3.500000000000000000, -7.449340926099361937, 0.01814118441321387054 ) ) ;
#4140=CARTESIAN_POINT ( 'NONE',  ( 3.500000000000000000, -5.849340926099361404, 0.01814118441321387054 ) ) ;
#4143=CARTESIAN_POINT ( 'NONE',  ( 2.815599370228907716, -0.7506590739006385737, -2.841254879263473310 ) ) ;
#4151=CARTESIAN_POINT ( 'NONE',  ( 2.134148098076978251, -6.049340926099361582, -2.108492589042307408 ) ) ;
#4155=AXIS2_PLACEMENT_3D ( 'NONE', #8945, #4032, #6913 ) ;
#4156=PRODUCT ( 'spring', 'spring', '', ( #364 ) ) ;
#4165=CARTESIAN_POINT ( 'NONE',  ( -2.487701488670255312, -5.249340926099360871, 2.462045979635577808 ) ) ;
#4166=CARTESIAN_POINT ( 'NONE',  ( 4.000000000000000000, -5.849340926099360516, 0.01814118441321914063 ) ) ;
#4174=CARTESIAN_POINT ( 'NONE',  ( -4.000000000000000000, 0.2493409260993615095, 0.01814118441313491634 ) ) ;
#4184=CARTESIAN_POINT ( 'NONE',  ( -1.260781871532494103, -3.749340926099361315, 2.992485675378538712 ) ) ;
#4187=CARTESIAN_POINT ( 'NONE',  ( -1.638713065079245634, -4.850659073900639662, 4.007514324621432422 ) ) ;
#4191=CARTESIAN_POINT ( 'NONE',  ( -3.250000000000006661, -0.000000000000000000, 0.5527349658716841363 ) ) ;
#4196=CARTESIAN_POINT ( 'NONE',  ( 2.134148098076978251, -7.649340926099361226, -2.108492589042307408 ) ) ;
#4209=CARTESIAN_POINT ( 'NONE',  ( 3.500000000000000000, -4.249340926099360871, 0.01814118441321387054 ) ) ;
#4210=CARTESIAN_POINT ( 'NONE',  ( 3.492485675378536047, -5.749340926099363536, 1.467888652719046672 ) ) ;
#4219=CARTESIAN_POINT ( 'NONE',  ( 3.492485675378566690, -5.450659073900639306, -1.467888652718972287 ) ) ;
#4230=CARTESIAN_POINT ( 'NONE',  ( 3.007514324621463508, -7.549340926099361582, -1.224499502706076770 ) ) ;
#4234=CARTESIAN_POINT ( 'NONE',  ( -4.000000000000000000, -1.350659073900638552, 0.01814118441313491634 ) ) ;
#4241=CARTESIAN_POINT ( 'NONE',  ( -1.260781871532494103, -5.349340926099361404, 2.992485675378538712 ) ) ;
#4250=CARTESIAN_POINT ( 'NONE',  ( -1.971654945569944140, -3.316496963571793567E-17, 2.933326779092722436 ) ) ;
#4253=CARTESIAN_POINT ( 'NONE',  ( -3.500000000000000000, -3.449340926099361049, -0.01814118441321344033 ) ) ;
#4259=CARTESIAN_POINT ( 'NONE',  ( 2.462045979635629767, -3.950659073900639751, -2.487701488670203354 ) ) ;
#4269=CARTESIAN_POINT ( 'NONE',  ( 2.134148098076978251, -4.449340926099361937, -2.108492589042307408 ) ) ;
#4276=CARTESIAN_POINT ( 'NONE',  ( 2.841254879263473310, -1.950659073900638640, 2.815599370228907272 ) ) ;
#4284=CARTESIAN_POINT ( 'NONE',  ( 1.260781871532430598, -0.2506590739006394064, 2.992485675378564469 ) ) ;
#4289=SURFACE_STYLE_USAGE ( .BOTH. , #2194 ) ;
#4296=CARTESIAN_POINT ( 'NONE',  ( 3.507514324621465285, -5.949340926099361937, -1.431606283892619125 ) ) ;
#4297=ORIENTED_EDGE ( 'NONE', *, *, #1607, .T. ) ;
#4299=CARTESIAN_POINT ( 'NONE',  ( -1.431606283892693066, -6.450659073900639306, 3.507514324621434199 ) ) ;
#4303=ORIENTED_EDGE ( 'NONE', *, *, #885, .T. ) ;
#4307=CARTESIAN_POINT ( 'NONE',  ( -1.467888652718973619, -7.450659073900638418, -3.492485675378565801 ) ) ;
#4317=CARTESIAN_POINT ( 'NONE',  ( 3.007514324621463508, -5.949340926099362825, -1.224499502706076770 ) ) ;
#4320=CARTESIAN_POINT ( 'NONE',  ( 2.815599370228847320, -2.449340926099361049, 2.841254879263533262 ) ) ;
#4330=CARTESIAN_POINT ( 'NONE',  ( -3.007514324621463508, -6.749340926099361759, 1.224499502706077658 ) ) ;
#4342=CARTESIAN_POINT ( 'NONE',  ( 2.462045979635577364, -5.649340926099361226, 2.487701488670255312 ) ) ;
#4354=CARTESIAN_POINT ( 'NONE',  ( -3.507514324621434199, -4.450659073900639306, -1.431606283892695064 ) ) ;
#4365=CARTESIAN_POINT ( 'NONE',  ( 1.260781871532495657, -1.349340926099361626, -2.992485675378538268 ) ) ;
#4367=CARTESIAN_POINT ( 'NONE',  ( 1.674995433905601239, -4.549340926099363358, -3.992485675378532939 ) ) ;
#4370=DIRECTION ( 'NONE',  ( 0.000000000000000000, -0.9973637043974449279, -0.07256473765270717025 ) ) ;
#4377=CARTESIAN_POINT ( 'NONE',  ( -1.224499502706140497, -4.850659073900639662, 3.007514324621436863 ) ) ;
#4386=CARTESIAN_POINT ( 'NONE',  ( 2.487701488670255756, -2.849340926099361404, -2.462045979635577364 ) ) ;
#4390=CARTESIAN_POINT ( 'NONE',  ( -1.431606283892620235, -4.749340926099363536, -3.507514324621463953 ) ) ;
#4398=CARTESIAN_POINT ( 'NONE',  ( -1.674995433905599462, -0.5493409260993608045, 3.992485675378533383 ) ) ;
#4409=CARTESIAN_POINT ( 'NONE',  ( -3.000000000000000444, -2.950659073900639306, 0.01814118441314532468 ) ) ;
#4411=CARTESIAN_POINT ( 'NONE',  ( -1.638713065079163034, -3.149340926099360782, -4.007514324621466173 ) ) ;
#4423=CARTESIAN_POINT ( 'NONE',  ( -0.01814118441314477650, -4.150659073900639484, -3.000000000000000444 ) ) ;
#4429=CARTESIAN_POINT ( 'NONE',  ( -3.500000000000000000, -6.649340926099361226, -0.01814118441321344033 ) ) ;
#4430=CARTESIAN_POINT ( 'NONE',  ( -3.750000000000000000, 0.000000000000000000, -3.927886379372531234E-14 ) ) ;
#4442=CARTESIAN_POINT ( 'NONE',  ( 4.007514324621432422, -6.850659073900641438, 1.638713065079246078 ) ) ;
#4451=CARTESIAN_POINT ( 'NONE',  ( -2.992485675378538268, -8.149340926099366555, -1.260781871532495879 ) ) ;
#4454=CARTESIAN_POINT ( 'NONE',  ( -1.638713065079163034, -4.749340926099361759, -4.007514324621466173 ) ) ;
#4458=CARTESIAN_POINT ( 'NONE',  ( 3.500000000000000000, -2.649340926099361226, 0.01814118441321387054 ) ) ;
#4464=CARTESIAN_POINT ( 'NONE',  ( -2.841254879263533262, -6.849340926099361404, 2.815599370228847764 ) ) ;
#4468=CARTESIAN_POINT ( 'NONE',  ( 2.487701488670203354, -0.3506590739006389956, 2.462045979635629323 ) ) ;
#4477=CARTESIAN_POINT ( 'NONE',  ( -1.431606283892620235, -1.549340926099361138, -3.507514324621463953 ) ) ;
#4494=CARTESIAN_POINT ( 'NONE',  ( 1.674995433905515085, -3.450659073900638862, 3.992485675378568022 ) ) ;
#4505=CARTESIAN_POINT ( 'NONE',  ( -1.224499502706140497, -1.650659073900639484, 3.007514324621436863 ) ) ;
#4507=CARTESIAN_POINT ( 'NONE',  ( 4.007514324621469726, -1.149340926099360782, -1.638713065079161257 ) ) ;
#4512=CARTESIAN_POINT ( 'NONE',  ( -2.462045979635576920, -3.249340926099361315, -2.487701488670255756 ) ) ;
#4516=CARTESIAN_POINT ( 'NONE',  ( 4.000000000000000000, -5.849340926099360516, 0.01814118441321914063 ) ) ;
#4521=CARTESIAN_POINT ( 'NONE',  ( -3.000000000000000444, -4.550659073900638951, 0.01814118441314532468 ) ) ;
#4525=CARTESIAN_POINT ( 'NONE',  ( 3.492485675378566690, -3.850659073900639218, -1.467888652718972287 ) ) ;
#4528=CARTESIAN_POINT ( 'NONE',  ( 3.500000000000000000, -1.049340926099360916, 0.01814118441321387054 ) ) ;
#4538=CARTESIAN_POINT ( 'NONE',  ( 2.815599370228907716, -7.150659073900638596, -2.841254879263473310 ) ) ;
#4549=CARTESIAN_POINT ( 'NONE',  ( -2.134148098076932953, -2.750659073900639573, -2.108492589042352705 ) ) ;
#4554=CARTESIAN_POINT ( 'NONE',  ( -0.01814118441321365544, -3.849340926099361404, 3.500000000000000000 ) ) ;
#4559=CARTESIAN_POINT ( 'NONE',  ( -1.638713065079163034, -1.549340926099360916, -4.007514324621466173 ) ) ;
#4563=CARTESIAN_POINT ( 'NONE',  ( 3.000000000000000444, -3.750659073900639573, -0.01814118441314496039 ) ) ;
#4566=CARTESIAN_POINT ( 'NONE',  ( -2.487701488670202910, -2.750659073900639129, -2.462045979635629767 ) ) ;
#4572=CARTESIAN_POINT ( 'NONE',  ( -2.462045979635576920, -4.849340926099361404, -2.487701488670255756 ) ) ;
#4584=CARTESIAN_POINT ( 'NONE',  ( 2.815599370228907716, -3.950659073900640195, -2.841254879263473310 ) ) ;
#4595=CARTESIAN_POINT ( 'NONE',  ( -0.01814118441314477650, -4.150659073900639484, -3.000000000000000444 ) ) ;
#4600=CARTESIAN_POINT ( 'NONE',  ( 1.467888652719048226, -2.949340926099361049, -3.492485675378535603 ) ) ;
#4605=CARTESIAN_POINT ( 'NONE',  ( 0.01814118441321938349, -7.849340926099360516, -4.000000000000000000 ) ) ;
#4608=CIRCLE ( 'NONE', #4155, 0.2499999999999998335 ) ;
#4610=CARTESIAN_POINT ( 'NONE',  ( -2.462045979635629323, -1.550659073900639173, 2.487701488670203798 ) ) ;
#4613=CARTESIAN_POINT ( 'NONE',  ( 2.462045979635629767, -0.7506590739006389068, -2.487701488670203354 ) ) ;
#4619=CARTESIAN_POINT ( 'NONE',  ( -2.134148098076978251, -0.4493409260993615484, 2.108492589042307408 ) ) ;
#4640=CARTESIAN_POINT ( 'NONE',  ( 3.500000000000000000, -2.150659073900639040, -0.01814118441313969030 ) ) ;
#4644=CARTESIAN_POINT ( 'NONE',  ( 2.462045979635577364, -2.449340926099361049, 2.487701488670255312 ) ) ;
#4650=CARTESIAN_POINT ( 'NONE',  ( -1.260781871532494103, -0.5493409260993613596, 2.992485675378538712 ) ) ;
#4652=CARTESIAN_POINT ( 'NONE',  ( 1.431606283892694842, -2.450659073900638862, -3.507514324621434199 ) ) ;
#4665=CARTESIAN_POINT ( 'NONE',  ( -2.992485675378538268, -1.749340926099361981, -1.260781871532495879 ) ) ;
#4679=CARTESIAN_POINT ( 'NONE',  ( -4.000000000000000000, -5.049340926099361582, -0.01814118441321865144 ) ) ;
#4686=CARTESIAN_POINT ( 'NONE',  ( 2.992485675378565357, -7.050659073900639839, -1.260781871532430376 ) ) ;
#4695=CARTESIAN_POINT ( 'NONE',  ( 2.992485675378538712, -0.9493409260993616039, 1.260781871532494103 ) ) ;
#4699=CARTESIAN_POINT ( 'NONE',  ( 3.507514324621434199, -5.250659073900640905, 1.431606283892693066 ) ) ;
#4704=CARTESIAN_POINT ( 'NONE',  ( -1.467888652718973841, -2.650659073900639040, -3.492485675378565801 ) ) ;
#4710=CARTESIAN_POINT ( 'NONE',  ( 2.108492589042307408, -2.449340926099361937, 2.134148098076978251 ) ) ;
#4723=CARTESIAN_POINT ( 'NONE',  ( -2.841254879263533262, -6.849340926099361404, 2.815599370228847764 ) ) ;
#4731=CARTESIAN_POINT ( 'NONE',  ( 3.507514324621434199, -2.050659073900638951, 1.431606283892693066 ) ) ;
#4739=CARTESIAN_POINT ( 'NONE',  ( 2.462045979635577364, -5.649340926099361226, 2.487701488670255312 ) ) ;
#4742=CARTESIAN_POINT ( 'NONE',  ( 1.431606283892694842, -4.050659073900638951, -3.507514324621434199 ) ) ;
#4749=CARTESIAN_POINT ( 'NONE',  ( -1.431606283892693066, -4.850659073900639662, 3.507514324621434199 ) ) ;
#4756=CARTESIAN_POINT ( 'NONE',  ( 3.007514324621463508, -1.149340926099361448, -1.224499502706076770 ) ) ;
#4764=CARTESIAN_POINT ( 'NONE',  ( 0.000000000000000000, 0.000000000000000000, 0.000000000000000000 ) ) ;
#4769=CARTESIAN_POINT ( 'NONE',  ( -2.487701488670255312, -0.4493409260993610488, 2.462045979635577808 ) ) ;
#4770=CARTESIAN_POINT ( 'NONE',  ( -1.674995433905599462, -5.349340926099361404, 3.992485675378533383 ) ) ;
#4779=CARTESIAN_POINT ( 'NONE',  ( -3.007514324621435531, -6.050659073900639839, -1.224499502706142273 ) ) ;
#4782=CARTESIAN_POINT ( 'NONE',  ( -3.492485675378535603, -6.549340926099361582, -1.467888652719048670 ) ) ;
#4787=CARTESIAN_POINT ( 'NONE',  ( -1.431606283892620235, -3.149340926099361671, -3.507514324621463953 ) ) ;
#4790=CARTESIAN_POINT ( 'NONE',  ( 3.992485675378568910, -5.450659073900638418, -1.674995433905514863 ) ) ;
#4799=CARTESIAN_POINT ( 'NONE',  ( 3.000000000000000444, -2.649340926099361671, 0.01814118441320859698 ) ) ;
#4813=CARTESIAN_POINT ( 'NONE',  ( -3.507514324621464397, -0.3493409260993610710, 1.431606283892619347 ) ) ;
#4814=CARTESIAN_POINT ( 'NONE',  ( 3.507514324621465285, -1.149340926099361226, -1.431606283892619125 ) ) ;
#4822=CARTESIAN_POINT ( 'NONE',  ( 3.500000000000000000, -0.5506590739006389512, -0.01814118441313969030 ) ) ;
#4830=CARTESIAN_POINT ( 'NONE',  ( -3.000000000000000444, -0.2493409260993614540, -0.01814118441320822922 ) ) ;
#4833=CARTESIAN_POINT ( 'NONE',  ( -2.841254879263473310, -5.950659073900640195, -2.815599370228907716 ) ) ;
#4840=CARTESIAN_POINT ( 'NONE',  ( 3.000000000000000444, -5.849340926099360516, 0.01814118441320859698 ) ) ;
#4849=FACE_OUTER_BOUND ( 'NONE', #329, .T. ) ;
#4851=CARTESIAN_POINT ( 'NONE',  ( 0.01814118441321408565, -4.649340926099361226, -3.500000000000000000 ) ) ;
#4852=CARTESIAN_POINT ( 'NONE',  ( -3.500000000000000000, -0.2493409260993610654, -0.01814118441321344033 ) ) ;
#4859=CARTESIAN_POINT ( 'NONE',  ( 1.674995433905515085, -0.2506590739006385182, 3.992485675378568022 ) ) ;
#4870=CARTESIAN_POINT ( 'NONE',  ( -2.134148098076978251, -6.849340926099361404, 2.108492589042307408 ) ) ;
#4874=CARTESIAN_POINT ( 'NONE',  ( -4.007514324621431534, -4.450659073900638418, -1.638713065079248521 ) ) ;
#4882=CARTESIAN_POINT ( 'NONE',  ( 1.260781871532495657, -7.749340926099362648, -2.992485675378538268 ) ) ;
#4886=MECHANICAL_DESIGN_GEOMETRIC_PRESENTATION_REPRESENTATION('',(#2525),#880);
#4894=CARTESIAN_POINT ( 'NONE',  ( -3.500000000000000000, -5.049340926099361582, -0.01814118441321344033 ) ) ;
#4895=CARTESIAN_POINT ( 'NONE',  ( 1.431606283892619125, -3.949340926099361049, 3.507514324621464397 ) ) ;
#4903=CARTESIAN_POINT ( 'NONE',  ( 3.992485675378568910, -0.6506590739006385959, -1.674995433905514863 ) ) ;
#4915=CARTESIAN_POINT ( 'NONE',  ( 2.992485675378538712, -7.349340926099363180, 1.260781871532494103 ) ) ;
#4919=CARTESIAN_POINT ( 'NONE',  ( 2.841254879263473310, -0.3506590739006385515, 2.815599370228907272 ) ) ;
#4922=EDGE_LOOP ( 'NONE', ( #9094, #1092 ) ) ;
#4925=CARTESIAN_POINT ( 'NONE',  ( 3.007514324621463508, -7.549340926099361582, -1.224499502706076770 ) ) ;
#4937=CARTESIAN_POINT ( 'NONE',  ( 1.431606283892619125, -0.7493409260993610932, 3.507514324621464397 ) ) ;
#4946=CARTESIAN_POINT ( 'NONE',  ( 0.01814118441313467001, -1.750659073900638685, 4.000000000000000000 ) ) ;
#4956=CARTESIAN_POINT ( 'NONE',  ( 2.108492589042307408, -5.649340926099361226, 2.134148098076978251 ) ) ;
#4959=CARTESIAN_POINT ( 'NONE',  ( 4.007514324621432422, -5.250659073900638241, 1.638713065079246078 ) ) ;
#4968=CARTESIAN_POINT ( 'NONE',  ( -0.01814118441320841310, -7.049340926099361582, 3.000000000000000444 ) ) ;
#4976=CARTESIAN_POINT ( 'NONE',  ( -3.121191317301271084, -3.932028342773297922E-17, 2.017464392153318187 ) ) ;
#4978=CARTESIAN_POINT ( 'NONE',  ( -3.500000000000000000, -6.649340926099361226, -0.01814118441321344033 ) ) ;
#4979=CARTESIAN_POINT ( 'NONE',  ( -2.462045979635576920, -8.049340926099361582, -2.487701488670255756 ) ) ;
#4986=CARTESIAN_POINT ( 'NONE',  ( -3.507514324621434199, -6.050659073900638951, -1.431606283892695064 ) ) ;
#4994=CARTESIAN_POINT ( 'NONE',  ( -3.492485675378536047, -1.749340926099361093, -1.467888652719048670 ) ) ;
#4996=CARTESIAN_POINT ( 'NONE',  ( -2.108492589042306964, -4.849340926099359628, -2.134148098076978251 ) ) ;
#5000=CARTESIAN_POINT ( 'NONE',  ( 1.638713065079161924, -3.949340926099361493, 4.007514324621467949 ) ) ;
#5009=CARTESIAN_POINT ( 'NONE',  ( 3.000000000000000444, -2.150659073900639484, -0.01814118441314496039 ) ) ;
#5022=CARTESIAN_POINT ( 'NONE',  ( -2.462045979635576920, -8.049340926099361582, -2.487701488670255756 ) ) ;
#5023=CARTESIAN_POINT ( 'NONE',  ( -3.507514324621464397, -5.149340926099360338, 1.431606283892619347 ) ) ;
#5026=CARTESIAN_POINT ( 'NONE',  ( 1.431606283892694620, -7.250659073900639129, -3.507514324621433754 ) ) ;
#5034=CARTESIAN_POINT ( 'NONE',  ( -2.462045979635629323, -4.750659073900639129, 2.487701488670203798 ) ) ;
#5046=CARTESIAN_POINT ( 'NONE',  ( -3.000000000000000444, -1.849340926099361404, -0.01814118441320822922 ) ) ;
#5049=CARTESIAN_POINT ( 'NONE',  ( -0.01814118441321889430, -0.6493409260993606713, 4.000000000000000000 ) ) ;
#5059=CARTESIAN_POINT ( 'NONE',  ( -2.462045979635629323, 0.04934092609936105434, 2.487701488670203798 ) ) ;
#5067=CARTESIAN_POINT ( 'NONE',  ( 3.492485675378536047, -4.149340926099361226, 1.467888652719046672 ) ) ;
#5072=CARTESIAN_POINT ( 'NONE',  ( -2.462045979635576920, -3.249340926099361315, -2.487701488670255756 ) ) ;
#5083=CARTESIAN_POINT ( 'NONE',  ( 3.992485675378568910, -2.250659073900638685, -1.674995433905514863 ) ) ;
#5096=CARTESIAN_POINT ( 'NONE',  ( 2.108492589042352705, -3.950659073900640195, -2.134148098076933397 ) ) ;
#5098=CARTESIAN_POINT ( 'NONE',  ( 4.000000000000000000, -2.649340926099360782, 0.01814118441321914063 ) ) ;
#5109=CARTESIAN_POINT ( 'NONE',  ( 2.134148098076933397, -6.750659073900640017, 2.108492589042352261 ) ) ;
#5115=PRODUCT_DEFINITION ( 'UNKNOWN', '', #2191, #7012 ) ;
#5117=CARTESIAN_POINT ( 'NONE',  ( -1.431606283892620235, -6.349340926099360516, -3.507514324621463953 ) ) ;
#5129=CARTESIAN_POINT ( 'NONE',  ( 2.841254879263473310, -5.150659073900639484, 2.815599370228907272 ) ) ;
#5130=ADVANCED_FACE ( 'NONE', ( #4849 ), #2950, .T. ) ;
#5140=CARTESIAN_POINT ( 'NONE',  ( 1.431606283892619125, -2.349340926099361848, 3.507514324621464397 ) ) ;
#5143=CARTESIAN_POINT ( 'NONE',  ( -1.224499502706140497, -0.05065907390063940224, 3.007514324621436863 ) ) ;
#5144=UNCERTAINTY_MEASURE_WITH_UNIT (LENGTH_MEASURE( 1.000000000000000082E-05 ), #5512, 'distance_accuracy_value', 'NONE');
#5146=CARTESIAN_POINT ( 'NONE',  ( 2.841254879263533262, -4.449340926099361937, -2.815599370228847320 ) ) ;
#5154=CARTESIAN_POINT ( 'NONE',  ( 0.01814118441321938349, -3.049340926099361138, -4.000000000000000000 ) ) ;
#5156=ORIENTED_EDGE ( 'NONE', *, *, #3316, .F. ) ;
#5159=CARTESIAN_POINT ( 'NONE',  ( 0.01814118441314514080, -6.550659073900640728, 3.000000000000000444 ) ) ;
#5167=CARTESIAN_POINT ( 'NONE',  ( -3.507514324621464397, -5.149340926099360338, 1.431606283892619347 ) ) ;
#5173=DIRECTION ( 'NONE',  ( 0.000000000000000000, 0.9973637043974448169, 0.07256473765270717025 ) ) ;
#5180=CARTESIAN_POINT ( 'NONE',  ( 4.000000000000000000, -3.750659073900638685, -0.01814118441313441674 ) ) ;
#5191=CARTESIAN_POINT ( 'NONE',  ( 0.01814118441320878086, -7.849340926099363180, -3.000000000000000444 ) ) ;
#5194=CARTESIAN_POINT ( 'NONE',  ( 0.01814118441321938349, -3.049340926099361138, -4.000000000000000000 ) ) ;
#5198=CARTESIAN_POINT ( 'NONE',  ( 3.492485675378535603, -0.9493409260993610488, 1.467888652719046672 ) ) ;
#5203=CARTESIAN_POINT ( 'NONE',  ( -1.638713065079163034, -4.749340926099361759, -4.007514324621466173 ) ) ;
#5207=CARTESIAN_POINT ( 'NONE',  ( -3.000000000000000444, -7.750659073900639129, 0.01814118441314532468 ) ) ;
#5209=ORIENTED_EDGE ( 'NONE', *, *, #3316, .T. ) ;
#5216=CARTESIAN_POINT ( 'NONE',  ( -0.01814118441321365544, -0.6493409260993610044, 3.500000000000000000 ) ) ;
#5227=CARTESIAN_POINT ( 'NONE',  ( -4.007514324621431534, -4.450659073900638418, -1.638713065079248521 ) ) ;
#5238=CARTESIAN_POINT ( 'NONE',  ( 2.992485675378565357, -5.450659073900638418, -1.260781871532430376 ) ) ;
#5240=AXIS2_PLACEMENT_3D ( 'NONE', #8136, #6544, #266 ) ;
#5244=CARTESIAN_POINT ( 'NONE',  ( -2.462045979635576920, -1.649340926099361004, -2.487701488670255756 ) ) ;
#5249=CARTESIAN_POINT ( 'NONE',  ( 4.007514324621469726, -7.549340926099361582, -1.638713065079161257 ) ) ;
#5253=CARTESIAN_POINT ( 'NONE',  ( -2.487701488670202910, -1.150659073900638818, -2.462045979635629767 ) ) ;
#5256=CARTESIAN_POINT ( 'NONE',  ( 3.500000000000000000, -0.5506590739006389512, -0.01814118441313969030 ) ) ;
#5262=CARTESIAN_POINT ( 'NONE',  ( -2.462045979635576920, -1.649340926099361004, -2.487701488670255756 ) ) ;
#5275=CARTESIAN_POINT ( 'NONE',  ( 4.000000000000000000, -6.950659073900639306, -0.01814118441313441674 ) ) ;
#5284=CARTESIAN_POINT ( 'NONE',  ( -2.108492589042352261, 0.04934092609936062412, 2.134148098076933397 ) ) ;
#5288=CARTESIAN_POINT ( 'NONE',  ( -2.487701488670255312, -2.049340926099361582, 2.462045979635577808 ) ) ;
#5292=CARTESIAN_POINT ( 'NONE',  ( -1.638713065079163034, -6.349340926099361404, -4.007514324621466173 ) ) ;
#5296=CARTESIAN_POINT ( 'NONE',  ( -2.462045979635629323, -6.350659073900638774, 2.487701488670203798 ) ) ;
#5299=CARTESIAN_POINT ( 'NONE',  ( -3.500000000000000000, -1.350659073900638996, 0.01814118441314012051 ) ) ;
#5306=CARTESIAN_POINT ( 'NONE',  ( -1.224499502706077880, -1.549340926099361804, -3.007514324621463064 ) ) ;
#5311=CARTESIAN_POINT ( 'NONE',  ( -1.930746022523279315, -1.460316824068202362E-13, 2.881131468811274576 ) ) ;
#5320=AXIS2_PLACEMENT_3D ( 'NONE', #4764, #1094, #341 ) ;
#5327=CARTESIAN_POINT ( 'NONE',  ( -3.007514324621435531, -7.650659073900639484, -1.224499502706142273 ) ) ;
#5340=CARTESIAN_POINT ( 'NONE',  ( -4.007514324621467949, -5.149340926099361226, 1.638713065079161924 ) ) ;
#5343=CARTESIAN_POINT ( 'NONE',  ( -0.01814118441313947866, -4.150659073900639484, -3.500000000000000000 ) ) ;
#5347=PLANE ( 'NONE',  #156 ) ;
#5354=CARTESIAN_POINT ( 'NONE',  ( -2.108492589042306964, -3.249340926099361759, -2.134148098076978251 ) ) ;
#5359=CARTESIAN_POINT ( 'NONE',  ( -3.250000000000000444, 0.000000000000000000, -3.404030812060692501E-14 ) ) ;
#5369=CARTESIAN_POINT ( 'NONE',  ( -1.467888652719046449, -2.149340926099360782, 3.492485675378536047 ) ) ;
#5377=CARTESIAN_POINT ( 'NONE',  ( 2.462045979635629767, -0.7506590739006389068, -2.487701488670203354 ) ) ;
#5387=CARTESIAN_POINT ( 'NONE',  ( 1.431606283892619125, -5.549340926099361582, 3.507514324621464397 ) ) ;
#5390=CARTESIAN_POINT ( 'NONE',  ( -3.507514324621434199, -7.650659073900639484, -1.431606283892695064 ) ) ;
#5394=CARTESIAN_POINT ( 'NONE',  ( 1.431606283892694620, -4.050659073900638951, -3.507514324621433754 ) ) ;
#5402=CARTESIAN_POINT ( 'NONE',  ( -3.000000000000000444, -1.849340926099361404, -0.01814118441320822922 ) ) ;
#5416=CARTESIAN_POINT ( 'NONE',  ( 2.841254879263533262, -7.649340926099361226, -2.815599370228847320 ) ) ;
#5424=CARTESIAN_POINT ( 'NONE',  ( -3.500000000000000000, -2.950659073900639306, 0.01814118441314012051 ) ) ;
#5435=CARTESIAN_POINT ( 'NONE',  ( 3.492485675378536047, -7.349340926099362292, 1.467888652719046672 ) ) ;
#5438=CARTESIAN_POINT ( 'NONE',  ( -3.500000000000000000, -2.950659073900639306, 0.01814118441314012051 ) ) ;
#5443=CARTESIAN_POINT ( 'NONE',  ( 1.431606283892694620, -2.450659073900638862, -3.507514324621433754 ) ) ;
#5450=CARTESIAN_POINT ( 'NONE',  ( -0.01814118441320841310, -2.249340926099360871, 3.000000000000000444 ) ) ;
#5459=FACE_OUTER_BOUND ( 'NONE', #2206, .T. ) ;
#5463=CARTESIAN_POINT ( 'NONE',  ( 3.507514324621465285, -5.949340926099361937, -1.431606283892619125 ) ) ;
#5464=CARTESIAN_POINT ( 'NONE',  ( -3.992485675378532939, -6.549340926099361582, -1.674995433905601683 ) ) ;
#5472=CARTESIAN_POINT ( 'NONE',  ( -2.462045979635629323, 0.04934092609936105434, 2.487701488670203798 ) ) ;
#5477=CIRCLE ( 'NONE', #1462, 0.2499999999999998335 ) ;
#5482=CARTESIAN_POINT ( 'NONE',  ( 0.01814118441321408565, -7.849340926099360516, -3.500000000000000000 ) ) ;
#5486=CARTESIAN_POINT ( 'NONE',  ( 1.467888652718972731, -3.450659073900638862, 3.492485675378566246 ) ) ;
#5490=CARTESIAN_POINT ( 'NONE',  ( -3.492485675378566246, -4.650659073900639484, 1.467888652718973175 ) ) ;
#5498=CARTESIAN_POINT ( 'NONE',  ( 1.260781871532495657, -1.349340926099361626, -2.992485675378538268 ) ) ;
#5503=B_SPLINE_CURVE_WITH_KNOTS ( 'NONE', 3,
 ( #5359, #4191, #8423, #7554, #7023, #650, #1180, #4024, #1090, #1791, #6011, #3932, #6859, #5311, #8849, #2052, #5967, #3327 ),
 .UNSPECIFIED., .F., .F.,
 ( 4, 2, 2, 2, 2, 2, 2, 2, 4 ),
 ( 0.000000000000000000, 0.001653989080654771947, 0.002480983620982158029, 0.002894480891145850745, 0.003101229526227697320, 0.003204603843768620824, 0.003256291002539082359, 0.003282134581924312476, 0.003307978161309543027 ),
 .UNSPECIFIED. ) ;
#5512=( LENGTH_UNIT ( ) NAMED_UNIT ( * ) SI_UNIT ( .MILLI., .METRE. ) );
#5514=CARTESIAN_POINT ( 'NONE',  ( -3.507514324621464397, -1.949340926099361271, 1.431606283892619347 ) ) ;
#5515=CARTESIAN_POINT ( 'NONE',  ( 4.007514324621469726, -5.949340926099362825, -1.638713065079161257 ) ) ;
#5522=CARTESIAN_POINT ( 'NONE',  ( -1.260781871532431708, -7.450659073900640195, -2.992485675378564469 ) ) ;
#5528=CARTESIAN_POINT ( 'NONE',  ( 0.01814118441321408565, -7.849340926099360516, -3.500000000000000000 ) ) ;
#5533=CARTESIAN_POINT ( 'NONE',  ( -2.487701488670255312, -6.849340926099361404, 2.462045979635577808 ) ) ;
#5534=CARTESIAN_POINT ( 'NONE',  ( -3.500000000000000000, -0.2493409260993610654, -0.01814118441321343686 ) ) ;
#5536=CARTESIAN_POINT ( 'NONE',  ( 1.674995433905515085, -5.050659073900638951, 3.992485675378568022 ) ) ;
#5543=CARTESIAN_POINT ( 'NONE',  ( -2.992485675378538268, -8.149340926099366555, -1.260781871532495879 ) ) ;
#5554=CARTESIAN_POINT ( 'NONE',  ( -1.925759277493323207, -9.035843541029837430E-14, 2.922632427747480222 ) ) ;
#5556=CARTESIAN_POINT ( 'NONE',  ( -1.467888652719046449, -3.749340926099360871, 3.492485675378536047 ) ) ;
#5557=CARTESIAN_POINT ( 'NONE',  ( 4.007514324621469726, -7.549340926099361582, -1.638713065079161257 ) ) ;
#5564=CARTESIAN_POINT ( 'NONE',  ( -3.500000000000000000, -6.150659073900639484, 0.01814118441314012051 ) ) ;
#5569=CARTESIAN_POINT ( 'NONE',  ( 2.487701488670255756, -6.049340926099361582, -2.462045979635577364 ) ) ;
#5573=CARTESIAN_POINT ( 'NONE',  ( 3.500000000000000000, -7.449340926099361937, 0.01814118441321387054 ) ) ;
#5577=CARTESIAN_POINT ( 'NONE',  ( 2.815599370228907716, -3.950659073900640195, -2.841254879263473310 ) ) ;
#5585=CARTESIAN_POINT ( 'NONE',  ( -1.260781871532431708, -2.650659073900639928, -2.992485675378564469 ) ) ;
#5597=CARTESIAN_POINT ( 'NONE',  ( -1.431606283892620235, -1.549340926099361138, -3.507514324621463953 ) ) ;
#5598=CARTESIAN_POINT ( 'NONE',  ( 2.462045979635577364, -4.049340926099360694, 2.487701488670255312 ) ) ;
#5605=CARTESIAN_POINT ( 'NONE',  ( -4.007514324621431534, -1.250659073900638685, -1.638713065079248521 ) ) ;
#5615=CARTESIAN_POINT ( 'NONE',  ( 0.01814118441320878086, -1.449340926099361493, -3.000000000000000444 ) ) ;
#5619=CARTESIAN_POINT ( 'NONE',  ( 4.007514324621432422, -0.4506590739006384738, 1.638713065079246078 ) ) ;
#5628=CARTESIAN_POINT ( 'NONE',  ( -2.108492589042352261, 0.04934092609936062412, 2.134148098076933397 ) ) ;
#5640=CARTESIAN_POINT ( 'NONE',  ( 2.462045979635577364, -5.649340926099361226, 2.487701488670255312 ) ) ;
#5650=CARTESIAN_POINT ( 'NONE',  ( 3.507514324621434199, -6.850659073900638774, 1.431606283892693066 ) ) ;
#5652=ORIENTED_EDGE ( 'NONE', *, *, #7383, .T. ) ;
#5662=CARTESIAN_POINT ( 'NONE',  ( 1.224499502706077214, -3.949340926099361493, 3.007514324621463508 ) ) ;
#5665=CARTESIAN_POINT ( 'NONE',  ( 0.01814118441313467001, -4.950659073900639306, 4.000000000000000000 ) ) ;
#5672=CARTESIAN_POINT ( 'NONE',  ( 0.01814118441314514080, -1.750659073900639351, 3.000000000000000444 ) ) ;
#5681=CARTESIAN_POINT ( 'NONE',  ( -2.281106635417135653, -1.535234168922110014E-16, 2.799845732222085992 ) ) ;
#5685=CARTESIAN_POINT ( 'NONE',  ( -2.487701488670255312, -5.249340926099360871, 2.462045979635577808 ) ) ;
#5694=CARTESIAN_POINT ( 'NONE',  ( -2.487701488670202910, -7.550659073900639839, -2.462045979635629767 ) ) ;
#5702=CARTESIAN_POINT ( 'NONE',  ( 3.507514324621465285, -1.149340926099361226, -1.431606283892619125 ) ) ;
#5703=CARTESIAN_POINT ( 'NONE',  ( -1.224499502706077880, -6.349340926099361404, -3.007514324621463064 ) ) ;
#5707=CARTESIAN_POINT ( 'NONE',  ( -2.815599370228907272, -1.550659073900638507, 2.841254879263473754 ) ) ;
#5716=CARTESIAN_POINT ( 'NONE',  ( 3.007514324621463508, -5.949340926099362825, -1.224499502706076770 ) ) ;
#5727=CARTESIAN_POINT ( 'NONE',  ( 0.01814118441321408565, -7.849340926099360516, -3.500000000000000000 ) ) ;
#5730=CARTESIAN_POINT ( 'NONE',  ( 1.467888652718972731, -6.650659073900639484, 3.492485675378566246 ) ) ;
#5737=CARTESIAN_POINT ( 'NONE',  ( 4.007514324621432422, -0.4506590739006384738, 1.638713065079246078 ) ) ;
#5749=CARTESIAN_POINT ( 'NONE',  ( -2.108492589042306964, -6.449340926099361049, -2.134148098076978251 ) ) ;
#5753=CARTESIAN_POINT ( 'NONE',  ( -2.841254879263533262, -3.649340926099360782, 2.815599370228847764 ) ) ;
#5755=DIRECTION ( 'NONE',  ( 1.039441819132096507E-14, 0.07256473765270715637, -0.9973637043974449279 ) ) ;
#5761=CARTESIAN_POINT ( 'NONE',  ( -0.01814118441314477650, -7.350659073900640550, -3.000000000000000444 ) ) ;
#5777=CARTESIAN_POINT ( 'NONE',  ( -2.487701488670202910, -5.950659073900639306, -2.462045979635629767 ) ) ;
#5785=CARTESIAN_POINT ( 'NONE',  ( 0.01814118441313467001, -4.950659073900639306, 4.000000000000000000 ) ) ;
#5798=CARTESIAN_POINT ( 'NONE',  ( 2.134148098076978251, -6.049340926099361582, -2.108492589042307408 ) ) ;
#5801=CARTESIAN_POINT ( 'NONE',  ( -1.674995433905516196, -7.450659073900640195, -3.992485675378566690 ) ) ;
#5813=CARTESIAN_POINT ( 'NONE',  ( 3.007514324621436863, -3.650659073900639928, 1.224499502706140719 ) ) ;
#5821=CARTESIAN_POINT ( 'NONE',  ( 3.507514324621465285, -5.949340926099361937, -1.431606283892619125 ) ) ;
#5827=CARTESIAN_POINT ( 'NONE',  ( -3.500000000000000000, -6.150659073900639484, 0.01814118441314012051 ) ) ;
#5835=CARTESIAN_POINT ( 'NONE',  ( 4.007514324621432422, -5.250659073900638241, 1.638713065079246078 ) ) ;
#5845=CARTESIAN_POINT ( 'NONE',  ( 2.992485675378565357, -2.250659073900640461, -1.260781871532430376 ) ) ;
#5847=CARTESIAN_POINT ( 'NONE',  ( -1.674995433905599462, -2.149340926099360782, 3.992485675378533383 ) ) ;
#5851=CARTESIAN_POINT ( 'NONE',  ( 3.492485675378535603, -5.749340926099362648, 1.467888652719046672 ) ) ;
#5855=CARTESIAN_POINT ( 'NONE',  ( -4.007514324621467949, -6.749340926099361759, 1.638713065079161924 ) ) ;
#5859=CARTESIAN_POINT ( 'NONE',  ( -3.007514324621435531, -6.050659073900639839, -1.224499502706142273 ) ) ;
#5866=CARTESIAN_POINT ( 'NONE',  ( -0.01814118441321365544, -2.249340926099361315, 3.500000000000000000 ) ) ;
#5869=CARTESIAN_POINT ( 'NONE',  ( 3.507514324621465285, -7.549340926099362470, -1.431606283892619125 ) ) ;
#5881=CARTESIAN_POINT ( 'NONE',  ( -3.992485675378568022, -4.650659073900640372, 1.674995433905515529 ) ) ;
#5890=CARTESIAN_POINT ( 'NONE',  ( 0.01814118441314514080, -1.750659073900639351, 3.000000000000000444 ) ) ;
#5893=CARTESIAN_POINT ( 'NONE',  ( -3.992485675378532939, -1.749340926099360871, -1.674995433905601683 ) ) ;
#5896=CARTESIAN_POINT ( 'NONE',  ( 3.507514324621465285, -4.349340926099361404, -1.431606283892619347 ) ) ;
#5901=CARTESIAN_POINT ( 'NONE',  ( 4.007514324621469726, -4.349340926099361404, -1.638713065079161257 ) ) ;
#5905=CARTESIAN_POINT ( 'NONE',  ( -3.000000000000000444, -6.150659073900639484, 0.01814118441314532468 ) ) ;
#5913=CARTESIAN_POINT ( 'NONE',  ( 1.431606283892619125, -0.7493409260993610932, 3.507514324621464397 ) ) ;
#5927=CARTESIAN_POINT ( 'NONE',  ( -4.000000000000000000, -6.150659073900637708, 0.01814118441313491634 ) ) ;
#5938=CARTESIAN_POINT ( 'NONE',  ( 3.000000000000000444, -5.350659073900639662, -0.01814118441314496039 ) ) ;
#5942=CARTESIAN_POINT ( 'NONE',  ( -0.01814118441321365544, -2.249340926099361315, 3.500000000000000000 ) ) ;
#5949=CARTESIAN_POINT ( 'NONE',  ( 2.815599370228847320, -7.249340926099360871, 2.841254879263533262 ) ) ;
#5953=CARTESIAN_POINT ( 'NONE',  ( -2.992485675378564469, -6.250659073900639129, 1.260781871532430820 ) ) ;
#5956=CARTESIAN_POINT ( 'NONE',  ( 1.467888652718972731, -0.2506590739006389623, 3.492485675378566246 ) ) ;
#5962=CARTESIAN_POINT ( 'NONE',  ( 1.431606283892619125, -3.949340926099361049, 3.507514324621464397 ) ) ;
#5967=CARTESIAN_POINT ( 'NONE',  ( -1.920924113947233058, -1.125130374610751609E-16, 2.915376471134273118 ) ) ;
#5971=CARTESIAN_POINT ( 'NONE',  ( 1.638713065079247855, -4.050659073900639839, -4.007514324621431534 ) ) ;
#5981=CARTESIAN_POINT ( 'NONE',  ( -1.224499502706077880, -7.949340926099362825, -3.007514324621463064 ) ) ;
#5986=DIRECTION ( 'NONE',  ( 1.000000000000000000, -0.000000000000000000, 1.047711134623677467E-14 ) ) ;
#5987=CARTESIAN_POINT ( 'NONE',  ( -3.500000000000000000, -5.049340926099361582, -0.01814118441321344033 ) ) ;
#5993=CARTESIAN_POINT ( 'NONE',  ( 1.638713065079161924, -5.549340926099361582, 4.007514324621467949 ) ) ;
#5997=CARTESIAN_POINT ( 'NONE',  ( 2.462045979635629767, -5.550659073900639839, -2.487701488670203354 ) ) ;
#6006=CARTESIAN_POINT ( 'NONE',  ( 2.134148098076978251, -4.449340926099361937, -2.108492589042307408 ) ) ;
#6007=FACE_OUTER_BOUND ( 'NONE', #4922, .T. ) ;
#6011=CARTESIAN_POINT ( 'NONE',  ( -1.984762707500143719, -4.474939649318853872E-16, 2.802807230515030668 ) ) ;
#6026=CARTESIAN_POINT ( 'NONE',  ( 2.134148098076933397, -6.750659073900640017, 2.108492589042352261 ) ) ;
#6029=CARTESIAN_POINT ( 'NONE',  ( -2.487701488670255312, -3.649340926099361226, 2.462045979635577808 ) ) ;
#6035=CARTESIAN_POINT ( 'NONE',  ( -3.992485675378532939, -4.949340926099361937, -1.674995433905601683 ) ) ;
#6039=CARTESIAN_POINT ( 'NONE',  ( -3.507514324621434199, -2.850659073900639662, -1.431606283892695064 ) ) ;
#6042=CARTESIAN_POINT ( 'NONE',  ( -2.462045979635629323, -6.350659073900638774, 2.487701488670203798 ) ) ;
#6044=CARTESIAN_POINT ( 'NONE',  ( 0.01814118441313990887, -3.350659073900639218, 3.500000000000000000 ) ) ;
#6050=CARTESIAN_POINT ( 'NONE',  ( -3.000000000000000444, -3.449340926099361493, -0.01814118441320822922 ) ) ;
#6051=DIRECTION ( 'NONE',  ( 1.039441819132097611E-14, 0.07256473765270715637, -0.9973637043974449279 ) ) ;
#6066=CARTESIAN_POINT ( 'NONE',  ( 4.000000000000000000, -4.249340926099360871, 0.01814118441321914063 ) ) ;
#6073=CARTESIAN_POINT ( 'NONE',  ( -1.260781871532431708, -5.850659073900641438, -2.992485675378564469 ) ) ;
#6078=CARTESIAN_POINT ( 'NONE',  ( 2.462045979635577364, -7.249340926099360871, 2.487701488670255312 ) ) ;
#6085=CARTESIAN_POINT ( 'NONE',  ( 1.467888652719048226, -6.149340926099360338, -3.492485675378536047 ) ) ;
#6090=CARTESIAN_POINT ( 'NONE',  ( -0.01814118441313947866, -2.550659073900638951, -3.500000000000000000 ) ) ;
#6096=CARTESIAN_POINT ( 'NONE',  ( -0.01814118441313947866, -4.150659073900639484, -3.500000000000000000 ) ) ;
#6103=CARTESIAN_POINT ( 'NONE',  ( 1.224499502706077214, -3.949340926099361493, 3.007514324621463508 ) ) ;
#6118=CARTESIAN_POINT ( 'NONE',  ( -2.815599370228846876, -8.049340926099359805, -2.841254879263533262 ) ) ;
#6126=CARTESIAN_POINT ( 'NONE',  ( 2.462045979635629767, -2.350659073900639218, -2.487701488670203354 ) ) ;
#6131=CARTESIAN_POINT ( 'NONE',  ( 1.467888652719048226, -7.749340926099361759, -3.492485675378535603 ) ) ;
#6138=CARTESIAN_POINT ( 'NONE',  ( 1.431606283892619125, -7.149340926099362115, 3.507514324621464397 ) ) ;
#6143=CARTESIAN_POINT ( 'NONE',  ( 3.492485675378566690, -2.250659073900639573, -1.467888652718972287 ) ) ;
#6154=CARTESIAN_POINT ( 'NONE',  ( 1.224499502706077214, -2.349340926099361848, 3.007514324621463508 ) ) ;
#6168=CARTESIAN_POINT ( 'NONE',  ( 3.507514324621465285, -4.349340926099361404, -1.431606283892619125 ) ) ;
#6169=CARTESIAN_POINT ( 'NONE',  ( -0.01814118441321889430, -7.049340926099361582, 4.000000000000000000 ) ) ;
#6177=CARTESIAN_POINT ( 'NONE',  ( -1.431606283892693066, -0.05065907390063895815, 3.507514324621434199 ) ) ;
#6182=CARTESIAN_POINT ( 'NONE',  ( 2.487701488670255756, -7.649340926099361226, -2.462045979635577364 ) ) ;
#6187=CARTESIAN_POINT ( 'NONE',  ( -0.01814118441321365544, -7.049340926099361582, 3.500000000000000000 ) ) ;
#6190=CARTESIAN_POINT ( 'NONE',  ( -3.492485675378566246, -1.450659073900639084, 1.467888652718973397 ) ) ;
#6194=CARTESIAN_POINT ( 'NONE',  ( 2.487701488670203354, -5.150659073900639484, 2.462045979635629323 ) ) ;
#6199=CARTESIAN_POINT ( 'NONE',  ( 1.431606283892619125, -7.149340926099362115, 3.507514324621464397 ) ) ;
#6213=CARTESIAN_POINT ( 'NONE',  ( 1.431606283892619125, -2.349340926099361848, 3.507514324621464397 ) ) ;
#6214=CARTESIAN_POINT ( 'NONE',  ( -0.01814118441321889430, -5.449340926099361937, 4.000000000000000000 ) ) ;
#6221=CARTESIAN_POINT ( 'NONE',  ( -2.134148098076932953, -7.550659073900640728, -2.108492589042352705 ) ) ;
#6225=CARTESIAN_POINT ( 'NONE',  ( -1.431606283892620235, -7.949340926099361049, -3.507514324621463953 ) ) ;
#6231=CARTESIAN_POINT ( 'NONE',  ( -1.467888652719046449, -5.349340926099361404, 3.492485675378536047 ) ) ;
#6235=CARTESIAN_POINT ( 'NONE',  ( 1.674995433905515085, -3.450659073900638862, 3.992485675378568022 ) ) ;
#6242=CARTESIAN_POINT ( 'NONE',  ( 2.108492589042352705, -0.7506590739006395729, -2.134148098076933397 ) ) ;
#6256=CARTESIAN_POINT ( 'NONE',  ( 3.500000000000000000, -1.049340926099360916, 0.01814118441321387054 ) ) ;
#6257=CARTESIAN_POINT ( 'NONE',  ( -4.000000000000000000, -6.649340926099362115, -0.01814118441321865144 ) ) ;
#6265=CARTESIAN_POINT ( 'NONE',  ( 2.841254879263473310, -1.950659073900638640, 2.815599370228907272 ) ) ;
#6272=CARTESIAN_POINT ( 'NONE',  ( -2.134148098076978251, -0.4493409260993615484, 2.108492589042307408 ) ) ;
#6276=CARTESIAN_POINT ( 'NONE',  ( -3.992485675378568022, -3.050659073900638951, 1.674995433905515529 ) ) ;
#6284=CARTESIAN_POINT ( 'NONE',  ( 1.224499502706142273, -2.450659073900639751, -3.007514324621435531 ) ) ;
#6296=CARTESIAN_POINT ( 'NONE',  ( 3.492485675378536047, -0.9493409260993610488, 1.467888652719046672 ) ) ;
#6304=CARTESIAN_POINT ( 'NONE',  ( 3.492485675378566690, -7.050659073900641616, -1.467888652718972287 ) ) ;
#6311=CARTESIAN_POINT ( 'NONE',  ( -1.925759277493323207, -9.035843541029837430E-14, 2.922632427747480222 ) ) ;
#6313=CARTESIAN_POINT ( 'NONE',  ( -1.260781871532494103, -6.949340926099362825, 2.992485675378538712 ) ) ;
#6316=CARTESIAN_POINT ( 'NONE',  ( -4.000000000000000000, -2.950659073900638862, 0.01814118441313491634 ) ) ;
#6323=CARTESIAN_POINT ( 'NONE',  ( 2.134148098076933397, -0.3506590739006394397, 2.108492589042352261 ) ) ;
#6333=CARTESIAN_POINT ( 'NONE',  ( -1.942253529302216952, 2.864554167741711444E-18, 2.933213925443324488 ) ) ;
#6335=CARTESIAN_POINT ( 'NONE',  ( 3.492485675378536047, -4.149340926099361226, 1.467888652719046672 ) ) ;
#6336=CARTESIAN_POINT ( 'NONE',  ( -3.492485675378536047, -4.949340926099361049, -1.467888652719048670 ) ) ;
#6345=CARTESIAN_POINT ( 'NONE',  ( -2.815599370228907272, 0.04934092609936149149, 2.841254879263473754 ) ) ;
#6355=CARTESIAN_POINT ( 'NONE',  ( 1.224499502706077214, -7.149340926099361226, 3.007514324621463508 ) ) ;
#6358=CARTESIAN_POINT ( 'NONE',  ( -4.007514324621431534, -2.850659073900638774, -1.638713065079248521 ) ) ;
#6366=CARTESIAN_POINT ( 'NONE',  ( -3.000000000000000444, 0.2493409260993606213, 0.01814118441314532468 ) ) ;
#6375=CARTESIAN_POINT ( 'NONE',  ( -2.214270216908088340, -1.191525181865939160E-11, 2.839183589524241658 ) ) ;
#6378=CARTESIAN_POINT ( 'NONE',  ( -3.492485675378536047, -6.549340926099363358, -1.467888652719048670 ) ) ;
#6387=ORIENTED_EDGE ( 'NONE', *, *, #1607, .F. ) ;
#6389=CARTESIAN_POINT ( 'NONE',  ( 1.467888652718972731, -6.650659073900639484, 3.492485675378566246 ) ) ;
#6398=CARTESIAN_POINT ( 'NONE',  ( -3.507514324621464397, -1.949340926099361271, 1.431606283892619347 ) ) ;
#6401=CARTESIAN_POINT ( 'NONE',  ( -3.007514324621463508, -1.949340926099361493, 1.224499502706077658 ) ) ;
#6404=CARTESIAN_POINT ( 'NONE',  ( 1.674995433905515085, -1.850659073900638774, 3.992485675378568022 ) ) ;
#6411=CARTESIAN_POINT ( 'NONE',  ( -2.992485675378564469, 0.1493409260993606713, 1.260781871532430820 ) ) ;
#6421=CARTESIAN_POINT ( 'NONE',  ( -3.750000000000000000, 0.000000000000000000, -3.927886379372531234E-14 ) ) ;
#6425=CARTESIAN_POINT ( 'NONE',  ( 2.462045979635577364, -7.249340926099360871, 2.487701488670255312 ) ) ;
#6434=CARTESIAN_POINT ( 'NONE',  ( 1.431606283892694842, -5.650659073900638596, -3.507514324621434199 ) ) ;
#6445=CARTESIAN_POINT ( 'NONE',  ( -1.260781871532494103, -5.349340926099361404, 2.992485675378538712 ) ) ;
#6446=DIRECTION ( 'NONE',  ( 1.039441819132096507E-14, 0.07256473765270715637, -0.9973637043974449279 ) ) ;
#6448=CARTESIAN_POINT ( 'NONE',  ( 1.674995433905515085, -6.650659073900639484, 3.992485675378568022 ) ) ;
#6456=CARTESIAN_POINT ( 'NONE',  ( -2.108492589042352261, -6.350659073900638774, 2.134148098076933397 ) ) ;
#6469=CARTESIAN_POINT ( 'NONE',  ( 1.431606283892619125, -5.549340926099361582, 3.507514324621464397 ) ) ;
#6479=CARTESIAN_POINT ( 'NONE',  ( 2.815599370228907716, -2.350659073900638774, -2.841254879263473310 ) ) ;
#6487=CARTESIAN_POINT ( 'NONE',  ( -1.431606283892620235, -1.549340926099361138, -3.507514324621463953 ) ) ;
#6489=CARTESIAN_POINT ( 'NONE',  ( -2.108492589042306964, -1.649340926099361448, -2.134148098076978251 ) ) ;
#6493=CARTESIAN_POINT ( 'NONE',  ( -2.815599370228846876, -4.849340926099359628, -2.841254879263533262 ) ) ;
#6501=CARTESIAN_POINT ( 'NONE',  ( -3.007514324621435531, -4.450659073900640195, -1.224499502706142273 ) ) ;
#6508=( NAMED_UNIT ( * ) SI_UNIT ( $, .STERADIAN. ) SOLID_ANGLE_UNIT ( ) );
#6512=CARTESIAN_POINT ( 'NONE',  ( -2.487701488670255312, -5.249340926099360871, 2.462045979635577808 ) ) ;
#6515=CARTESIAN_POINT ( 'NONE',  ( -3.507514324621464397, -6.749340926099361759, 1.431606283892619347 ) ) ;
#6516=( BOUNDED_CURVE ( )  B_SPLINE_CURVE ( 2, ( #1825, #280, #1025, #5956, #7402, #2625, #5256, #420, #4613, #8102, #3875, #979, #1170, #4013, #5299, #8839, #8976, #2576, #7499, #6794, #8197, #8150, #1729, #3920, #6848, #5443, #6747, #4704, #4566, #2476, #3825, #1778, #7452, #6651, #6044, #8289, #470, #8880, #3266, #4525, #1126, #5394, #6096, #8245, #8795, #2668, #7594, #5490, #1922, #4749, #1219, #4059, #6194, #6895, #522, #3364, #9022, #804, #7221, #758, #5777, #2913, #5827, #6568, #6042, #4299, #2299, #5730, #155, #203, #897, #6520, #1454, #5026, #1551, #8879, #2522, #6745, #8619 ),
 .UNSPECIFIED., .F., .F. ) 
 B_SPLINE_CURVE_WITH_KNOTS ( ( 3, 2, 2, 2, 2, 2, 2, 2, 2, 2, 2, 2, 2, 2, 2, 2, 2, 2, 2, 2, 2, 2, 2, 2, 2, 2, 2, 2, 2, 2, 2, 2, 2, 2, 2, 2, 2, 2, 2, 3 ),
 ( 0.03135029301116579181, 0.05000000000000000278, 0.07499999999999999722, 0.1000000000000000056, 0.1250000000000000000, 0.1499999999999999944, 0.1749999999999999889, 0.2000000000000000111, 0.2250000000000000056, 0.2500000000000000000, 0.2750000000000000222, 0.2999999999999999334, 0.3249999999999999556, 0.3499999999999999778, 0.3750000000000000000, 0.4000000000000000222, 0.4249999999999999334, 0.4499999999999999556, 0.4749999999999999778, 0.5000000000000000000, 0.5250000000000000222, 0.5500000000000000444, 0.5749999999999999556, 0.5999999999999999778, 0.6250000000000000000, 0.6499999999999999112, 0.6750000000000000444, 0.6999999999999999556, 0.7249999999999999778, 0.7500000000000000000, 0.7750000000000000222, 0.8000000000000000444, 0.8249999999999999556, 0.8499999999999999778, 0.8750000000000000000, 0.8999999999999999112, 0.9250000000000000444, 0.9499999999999999556, 0.9749999999999999778, 1.000000000000000000 ),
 .UNSPECIFIED. ) 
 CURVE ( )  GEOMETRIC_REPRESENTATION_ITEM ( )  RATIONAL_B_SPLINE_CURVE ( ( 0.9711519008064275482, 0.9432150234192966387, 1.000000000000000000, 0.9238795325112867385, 1.000000000000000000, 0.9238795325112867385, 1.000000000000000000, 0.9238795325112867385, 1.000000000000000000, 0.9238795325112867385, 1.000000000000000000, 0.9238795325112867385, 1.000000000000000000, 0.9238795325112867385, 1.000000000000000000, 0.9238795325112867385, 1.000000000000000000, 0.9238795325112867385, 1.000000000000000000, 0.9238795325112867385, 1.000000000000000000, 0.9238795325112867385, 1.000000000000000000, 0.9238795325112867385, 1.000000000000000000, 0.9238795325112867385, 1.000000000000000000, 0.9238795325112867385, 1.000000000000000000, 0.9238795325112867385, 1.000000000000000000, 0.9238795325112867385, 1.000000000000000000, 0.9238795325112867385, 1.000000000000000000, 0.9238795325112867385, 1.000000000000000000, 0.9238795325112867385, 1.000000000000000000, 0.9238795325112867385, 1.000000000000000000, 0.9238795325112867385, 1.000000000000000000, 0.9238795325112867385, 1.000000000000000000, 0.9238795325112867385, 1.000000000000000000, 0.9238795325112867385, 1.000000000000000000, 0.9238795325112867385, 1.000000000000000000, 0.9238795325112867385, 1.000000000000000000, 0.9238795325112867385, 1.000000000000000000, 0.9238795325112867385, 1.000000000000000000, 0.9238795325112867385, 1.000000000000000000, 0.9238795325112867385, 1.000000000000000000, 0.9238795325112867385, 1.000000000000000000, 0.9238795325112867385, 1.000000000000000000, 0.9238795325112867385, 1.000000000000000000, 0.9238795325112867385, 1.000000000000000000, 0.9238795325112867385, 1.000000000000000000, 0.9238795325112867385, 1.000000000000000000, 0.9238795325112867385, 1.000000000000000000, 0.9238795325112867385, 1.000000000000000000, 0.9238795325112867385, 1.000000000000000000 ) ) 
 REPRESENTATION_ITEM ( '' )  );
#6520=CARTESIAN_POINT ( 'NONE',  ( 3.492485675378566690, -7.050659073900639839, -1.467888652718972287 ) ) ;
#6527=CARTESIAN_POINT ( 'NONE',  ( 2.815599370228847320, -0.8493409260993607379, 2.841254879263533262 ) ) ;
#6536=CARTESIAN_POINT ( 'NONE',  ( -3.500000000000000000, -1.849340926099361182, -0.01814118441321344033 ) ) ;
#6538=CARTESIAN_POINT ( 'NONE',  ( -2.108492589042306964, -8.049340926099361582, -2.134148098076978251 ) ) ;
#6542=CARTESIAN_POINT ( 'NONE',  ( 2.815599370228847320, -4.049340926099360694, 2.841254879263533262 ) ) ;
#6544=DIRECTION ( 'NONE',  ( -1.044949058366720058E-14, -0.07256473765270715637, 0.9973637043974449279 ) ) ;
#6545=CARTESIAN_POINT ( 'NONE',  ( 2.487701488670255756, -4.449340926099361937, -2.462045979635577364 ) ) ;
#6551=CARTESIAN_POINT ( 'NONE',  ( -2.815599370228846876, -4.849340926099359628, -2.841254879263533262 ) ) ;
#6555=CARTESIAN_POINT ( 'NONE',  ( 0.01814118441314514080, -3.350659073900639662, 3.000000000000000444 ) ) ;
#6563=CARTESIAN_POINT ( 'NONE',  ( -1.467888652719046449, -6.949340926099361049, 3.492485675378536047 ) ) ;
#6568=CARTESIAN_POINT ( 'NONE',  ( -3.492485675378566246, -6.250659073900640017, 1.467888652718973175 ) ) ;
#6573=ORIENTED_EDGE ( 'NONE', *, *, #8365, .T. ) ;
#6578=CARTESIAN_POINT ( 'NONE',  ( 1.638713065079247855, -2.450659073900638862, -4.007514324621431534 ) ) ;
#6589=CARTESIAN_POINT ( 'NONE',  ( -2.462045979635576920, -1.649340926099361004, -2.487701488670255756 ) ) ;
#6591=CARTESIAN_POINT ( 'NONE',  ( 1.260781871532495657, -7.749340926099362648, -2.992485675378538268 ) ) ;
#6593=CARTESIAN_POINT ( 'NONE',  ( 2.815599370228847320, -0.8493409260993607379, 2.841254879263533262 ) ) ;
#6597=CARTESIAN_POINT ( 'NONE',  ( -0.01814118441321365544, -5.449340926099361937, 3.500000000000000000 ) ) ;
#6601=CARTESIAN_POINT ( 'NONE',  ( -1.638713065079163034, -3.149340926099360782, -4.007514324621466173 ) ) ;
#6605=CARTESIAN_POINT ( 'NONE',  ( 3.492485675378566690, -0.6506590739006391511, -1.467888652718972287 ) ) ;
#6611=CARTESIAN_POINT ( 'NONE',  ( -2.462045979635576920, -3.249340926099361315, -2.487701488670255756 ) ) ;
#6624=CARTESIAN_POINT ( 'NONE',  ( 0.01814118441313467001, -3.350659073900638774, 4.000000000000000000 ) ) ;
#6627=ADVANCED_FACE ( 'NONE', ( #5459 ), #6711, .T. ) ;
#6634=CARTESIAN_POINT ( 'NONE',  ( -2.108492589042352261, -4.750659073900640017, 2.134148098076933397 ) ) ;
#6638=CARTESIAN_POINT ( 'NONE',  ( 1.431606283892619347, -0.7493409260993610932, 3.507514324621464397 ) ) ;
#6643=CARTESIAN_POINT ( 'NONE',  ( -0.01814118441321889430, -5.449340926099361937, 4.000000000000000000 ) ) ;
#6647=CARTESIAN_POINT ( 'NONE',  ( -2.134148098076932953, -4.350659073900638774, -2.108492589042352705 ) ) ;
#6651=CARTESIAN_POINT ( 'NONE',  ( -1.431606283892693066, -3.250659073900639129, 3.507514324621434199 ) ) ;
#6655=CARTESIAN_POINT ( 'NONE',  ( 1.467888652719048226, -2.949340926099361493, -3.492485675378536047 ) ) ;
#6668=CARTESIAN_POINT ( 'NONE',  ( 3.992485675378568910, -5.450659073900638418, -1.674995433905514863 ) ) ;
#6680=CARTESIAN_POINT ( 'NONE',  ( -2.134148098076932953, -1.150659073900639040, -2.108492589042352705 ) ) ;
#6682=CARTESIAN_POINT ( 'NONE',  ( 2.487701488670255756, -2.849340926099361404, -2.462045979635577364 ) ) ;
#6688=CARTESIAN_POINT ( 'NONE',  ( 2.815599370228847320, -4.049340926099360694, 2.841254879263533262 ) ) ;
#6692=CARTESIAN_POINT ( 'NONE',  ( -3.507514324621434199, -6.050659073900638951, -1.431606283892695064 ) ) ;
#6703=CARTESIAN_POINT ( 'NONE',  ( 2.462045979635577364, -2.449340926099361049, 2.487701488670255312 ) ) ;
#6711=PLANE ( 'NONE',  #5320 ) ;
#6713=CARTESIAN_POINT ( 'NONE',  ( 2.841254879263533262, -1.249340926099360871, -2.815599370228847320 ) ) ;
#6723=CARTESIAN_POINT ( 'NONE',  ( -3.007514324621435531, -2.850659073900640106, -1.224499502706142273 ) ) ;
#6730=CARTESIAN_POINT ( 'NONE',  ( -1.431606283892620235, -1.549340926099361138, -3.507514324621463953 ) ) ;
#6735=CARTESIAN_POINT ( 'NONE',  ( -4.007514324621467949, -1.949340926099360827, 1.638713065079161924 ) ) ;
#6741=CARTESIAN_POINT ( 'NONE',  ( -3.492485675378566246, -4.650659073900639484, 1.467888652718973397 ) ) ;
#6745=CARTESIAN_POINT ( 'NONE',  ( -3.507514324621433754, -7.650659073900639484, -1.431606283892695064 ) ) ;
#6747=CARTESIAN_POINT ( 'NONE',  ( -0.01814118441313947866, -2.550659073900638951, -3.500000000000000000 ) ) ;
#6754=CARTESIAN_POINT ( 'NONE',  ( -1.431606283892620235, -7.949340926099361049, -3.507514324621463953 ) ) ;
#6767=CARTESIAN_POINT ( 'NONE',  ( 0.01814118441313467001, -6.550659073900640728, 4.000000000000000000 ) ) ;
#6775=CARTESIAN_POINT ( 'NONE',  ( -0.01814118441313947866, -0.9506590739006390844, -3.500000000000000000 ) ) ;
#6785=CARTESIAN_POINT ( 'NONE',  ( -1.467888652719046449, -3.749340926099360871, 3.492485675378536047 ) ) ;
#6788=CARTESIAN_POINT ( 'NONE',  ( 3.500000000000000000, -6.950659073900639306, -0.01814118441313969030 ) ) ;
#6794=CARTESIAN_POINT ( 'NONE',  ( 1.467888652718972731, -1.850659073900638996, 3.492485675378566246 ) ) ;
#6801=CARTESIAN_POINT ( 'NONE',  ( -2.462045979635576920, -8.049340926099361582, -2.487701488670255756 ) ) ;
#6809=CARTESIAN_POINT ( 'NONE',  ( 0.01814118441320878086, -3.049340926099361138, -3.000000000000000444 ) ) ;
#6817=CARTESIAN_POINT ( 'NONE',  ( -4.007514324621467949, -6.749340926099361759, 1.638713065079161924 ) ) ;
#6828=CARTESIAN_POINT ( 'NONE',  ( 3.492485675378566690, -2.250659073900639573, -1.467888652718972287 ) ) ;
#6839=CARTESIAN_POINT ( 'NONE',  ( 2.134148098076978251, -1.249340926099361537, -2.108492589042307408 ) ) ;
#6842=CARTESIAN_POINT ( 'NONE',  ( 3.500000000000000000, -2.150659073900639040, -0.01814118441313969030 ) ) ;
#6848=CARTESIAN_POINT ( 'NONE',  ( 2.462045979635629767, -2.350659073900639218, -2.487701488670203354 ) ) ;
#6854=CARTESIAN_POINT ( 'NONE',  ( 3.492485675378536047, -7.349340926099362292, 1.467888652719046672 ) ) ;
#6859=CARTESIAN_POINT ( 'NONE',  ( -1.943399160878812371, -1.460316824068199838E-13, 2.858293051873583845 ) ) ;
#6861=DIRECTION ( 'NONE',  ( 1.000000000000000000, 0.000000000000000000, 0.000000000000000000 ) ) ;
#6868=CARTESIAN_POINT ( 'NONE',  ( 2.462045979635577364, -0.8493409260993610710, 2.487701488670255312 ) ) ;
#6869=CARTESIAN_POINT ( 'NONE',  ( -0.01814118441321365544, -2.249340926099361315, 3.500000000000000000 ) ) ;
#6876=CARTESIAN_POINT ( 'NONE',  ( 0.01814118441313990887, -3.350659073900639218, 3.500000000000000000 ) ) ;
#6886=CARTESIAN_POINT ( 'NONE',  ( 2.487701488670255756, -4.449340926099361937, -2.462045979635577364 ) ) ;
#6890=CARTESIAN_POINT ( 'NONE',  ( 3.507514324621434199, -6.850659073900638774, 1.431606283892693066 ) ) ;
#6895=CARTESIAN_POINT ( 'NONE',  ( 3.507514324621434199, -5.250659073900640905, 1.431606283892693066 ) ) ;
#6903=CARTESIAN_POINT ( 'NONE',  ( -3.007514324621463508, -5.149340926099361226, 1.224499502706077658 ) ) ;
#6913=DIRECTION ( 'NONE',  ( 0.000000000000000000, -0.9973637043974449279, -0.07256473765270717025 ) ) ;
#6915=CARTESIAN_POINT ( 'NONE',  ( -2.487701488670255312, -3.649340926099361226, 2.462045979635577808 ) ) ;
#6916=CARTESIAN_POINT ( 'NONE',  ( -3.492485675378536047, -1.749340926099361093, -1.467888652719048670 ) ) ;
#6923=CARTESIAN_POINT ( 'NONE',  ( 2.487701488670203354, -0.3506590739006389956, 2.462045979635629323 ) ) ;
#6928=CARTESIAN_POINT ( 'NONE',  ( -3.492485675378535603, -8.149340926099361226, -1.467888652719048670 ) ) ;
#6931=CARTESIAN_POINT ( 'NONE',  ( 3.507514324621465285, -5.949340926099361937, -1.431606283892619125 ) ) ;
#6934=CARTESIAN_POINT ( 'NONE',  ( -0.01814118441313417734, -5.750659073900639129, -4.000000000000000000 ) ) ;
#6940=CARTESIAN_POINT ( 'NONE',  ( -1.260781871532494103, -2.149340926099361226, 2.992485675378538712 ) ) ;
#6953=CARTESIAN_POINT ( 'NONE',  ( 3.492485675378536047, -2.549340926099360694, 1.467888652719046672 ) ) ;
#6954=CARTESIAN_POINT ( 'NONE',  ( -4.007514324621467949, -5.149340926099361226, 1.638713065079161924 ) ) ;
#6962=CARTESIAN_POINT ( 'NONE',  ( -2.134148098076932953, -5.950659073900640195, -2.108492589042352705 ) ) ;
#6973=CARTESIAN_POINT ( 'NONE',  ( -1.467888652719046449, -6.949340926099361049, 3.492485675378536047 ) ) ;
#6976=CARTESIAN_POINT ( 'NONE',  ( -2.841254879263473310, -2.750659073900638685, -2.815599370228907716 ) ) ;
#6986=CARTESIAN_POINT ( 'NONE',  ( 1.260781871532430598, -1.850659073900639884, 2.992485675378564469 ) ) ;
#6996=CARTESIAN_POINT ( 'NONE',  ( -3.507514324621464397, -0.3493409260993610710, 1.431606283892619347 ) ) ;
#6999=CARTESIAN_POINT ( 'NONE',  ( -1.467888652719046449, -5.349340926099361404, 3.492485675378536047 ) ) ;
#7000=CARTESIAN_POINT ( 'NONE',  ( 2.462045979635577364, -0.8493409260993610710, 2.487701488670255312 ) ) ;
#7008=CARTESIAN_POINT ( 'NONE',  ( -3.492485675378566246, -4.650659073900639484, 1.467888652718973397 ) ) ;
#7012=PRODUCT_DEFINITION_CONTEXT ( 'detailed design', #3735, 'design' ) ;
#7016=CARTESIAN_POINT ( 'NONE',  ( 2.108492589042307408, -4.049340926099361582, 2.134148098076978251 ) ) ;
#7020=CARTESIAN_POINT ( 'NONE',  ( -2.841254879263473310, -4.350659073900638774, -2.815599370228907716 ) ) ;
#7023=CARTESIAN_POINT ( 'NONE',  ( -2.605717154052086038, -1.491716277579526044E-16, 2.068367651695531162 ) ) ;
#7031=CARTESIAN_POINT ( 'NONE',  ( 1.224499502706077214, -5.549340926099361582, 3.007514324621463508 ) ) ;
#7037=PRESENTATION_STYLE_ASSIGNMENT (( #4289 ) ) ;
#7043=CARTESIAN_POINT ( 'NONE',  ( -3.507514324621464397, -3.549340926099361582, 1.431606283892619347 ) ) ;
#7044=CARTESIAN_POINT ( 'NONE',  ( -2.487701488670255312, -3.649340926099361226, 2.462045979635577808 ) ) ;
#7051=CARTESIAN_POINT ( 'NONE',  ( -2.462045979635629323, -6.350659073900638774, 2.487701488670203798 ) ) ;
#7061=CARTESIAN_POINT ( 'NONE',  ( 2.134148098076978251, -7.649340926099361226, -2.108492589042307408 ) ) ;
#7064=CARTESIAN_POINT ( 'NONE',  ( 0.01814118441313467001, -1.750659073900638685, 4.000000000000000000 ) ) ;
#7072=CARTESIAN_POINT ( 'NONE',  ( 1.260781871532495657, -6.149340926099362115, -2.992485675378538268 ) ) ;
#7083=CARTESIAN_POINT ( 'NONE',  ( -2.000431855567539330, -3.316496963571793567E-17, 2.928653597410987075 ) ) ;
#7086=CARTESIAN_POINT ( 'NONE',  ( -2.462045979635576920, -4.849340926099361404, -2.487701488670255756 ) ) ;
#7093=CARTESIAN_POINT ( 'NONE',  ( 3.492485675378566690, -3.850659073900639218, -1.467888652718972287 ) ) ;
#7105=CARTESIAN_POINT ( 'NONE',  ( -2.992485675378538268, -4.949340926099361937, -1.260781871532495879 ) ) ;
#7108=CARTESIAN_POINT ( 'NONE',  ( -1.638713065079245634, -1.650659073900638818, 4.007514324621432422 ) ) ;
#7117=CARTESIAN_POINT ( 'NONE',  ( 0.01814118441314514080, -0.1506590739006394009, 3.000000000000000444 ) ) ;
#7134=CARTESIAN_POINT ( 'NONE',  ( 1.467888652719048226, -4.549340926099360694, -3.492485675378536047 ) ) ;
#7143=CARTESIAN_POINT ( 'NONE',  ( -3.500000000000000000, -7.750659073900639129, 0.01814118441314012051 ) ) ;
#7146=VERTEX_POINT ( 'NONE', #5534 ) ;
#7151=CARTESIAN_POINT ( 'NONE',  ( 3.500000000000000000, -1.049340926099360916, 0.01814118441321387054 ) ) ;
#7153=CARTESIAN_POINT ( 'NONE',  ( 2.134148098076978251, -2.849340926099362292, -2.108492589042307408 ) ) ;
#7156=CARTESIAN_POINT ( 'NONE',  ( 4.000000000000000000, -1.049340926099360916, 0.01814118441321914063 ) ) ;
#7163=CARTESIAN_POINT ( 'NONE',  ( -2.992485675378564469, -1.450659073900639751, 1.260781871532430820 ) ) ;
#7178=CARTESIAN_POINT ( 'NONE',  ( 3.507514324621465285, -7.549340926099362470, -1.431606283892619125 ) ) ;
#7189=CARTESIAN_POINT ( 'NONE',  ( 0.01814118441313990887, -4.950659073900639306, 3.500000000000000000 ) ) ;
#7195=CARTESIAN_POINT ( 'NONE',  ( 1.431606283892619125, -0.7493409260993610932, 3.507514324621464397 ) ) ;
#7198=CARTESIAN_POINT ( 'NONE',  ( 1.224499502706077214, -2.349340926099361848, 3.007514324621463508 ) ) ;
#7201=CARTESIAN_POINT ( 'NONE',  ( -1.638713065079245634, -6.450659073900638418, 4.007514324621432422 ) ) ;
#7209=CARTESIAN_POINT ( 'NONE',  ( 1.224499502706142273, -5.650659073900639484, -3.007514324621435531 ) ) ;
#7216=CARTESIAN_POINT ( 'NONE',  ( 0.01814118441321408565, -1.449340926099361271, -3.500000000000000000 ) ) ;
#7218=CARTESIAN_POINT ( 'NONE',  ( -0.01814118441321365544, -7.049340926099361582, 3.500000000000000000 ) ) ;
#7219=CARTESIAN_POINT ( 'NONE',  ( -3.500000000000000000, -5.049340926099361582, -0.01814118441321344033 ) ) ;
#7221=CARTESIAN_POINT ( 'NONE',  ( -0.01814118441313947866, -5.750659073900639129, -3.500000000000000000 ) ) ;
#7228=CARTESIAN_POINT ( 'NONE',  ( 0.01814118441313467001, -6.550659073900640728, 4.000000000000000000 ) ) ;
#7239=CARTESIAN_POINT ( 'NONE',  ( 1.224499502706142273, -4.050659073900639839, -3.007514324621435531 ) ) ;
#7242=CARTESIAN_POINT ( 'NONE',  ( -1.674995433905599462, -3.749340926099360871, 3.992485675378533383 ) ) ;
#7251=CARTESIAN_POINT ( 'NONE',  ( 1.674995433905601239, -6.149340926099362115, -3.992485675378532939 ) ) ;
#7255=CARTESIAN_POINT ( 'NONE',  ( 2.992485675378565357, -3.850659073900639662, -1.260781871532430376 ) ) ;
#7264=CARTESIAN_POINT ( 'NONE',  ( -3.507514324621464397, -6.749340926099361759, 1.431606283892619347 ) ) ;
#7279=CARTESIAN_POINT ( 'NONE',  ( -2.815599370228907272, -3.150659073900639040, 2.841254879263473754 ) ) ;
#7290=CARTESIAN_POINT ( 'NONE',  ( 0.01814118441314514080, -0.1506590739006394009, 3.000000000000000444 ) ) ;
#7293=CARTESIAN_POINT ( 'NONE',  ( -3.992485675378568022, -6.250659073900639129, 1.674995433905515529 ) ) ;
#7296=CARTESIAN_POINT ( 'NONE',  ( -3.507514324621464397, -3.549340926099361138, 1.431606283892619569 ) ) ;
#7302=CARTESIAN_POINT ( 'NONE',  ( -0.01814118441321889430, -7.049340926099361582, 4.000000000000000000 ) ) ;
#7306=CARTESIAN_POINT ( 'NONE',  ( 3.507514324621434199, -0.4506590739006390844, 1.431606283892693066 ) ) ;
#7315=CARTESIAN_POINT ( 'NONE',  ( -3.500000000000000000, -1.849340926099361182, -0.01814118441321344033 ) ) ;
#7325=CARTESIAN_POINT ( 'NONE',  ( 2.815599370228907716, -5.550659073900638063, -2.841254879263473310 ) ) ;
#7336=CARTESIAN_POINT ( 'NONE',  ( 2.134148098076933397, -3.550659073900639395, 2.108492589042352261 ) ) ;
#7338=CARTESIAN_POINT ( 'NONE',  ( -4.000000000000000000, -3.449340926099361049, -0.01814118441321865144 ) ) ;
#7341=CARTESIAN_POINT ( 'NONE',  ( -1.467888652719046449, -2.149340926099360782, 3.492485675378535603 ) ) ;
#7346=CARTESIAN_POINT ( 'NONE',  ( 1.674995433905601239, -2.949340926099360605, -3.992485675378532939 ) ) ;
#7350=CARTESIAN_POINT ( 'NONE',  ( 1.260781871532430598, -3.450659073900639751, 2.992485675378564469 ) ) ;
#7359=CARTESIAN_POINT ( 'NONE',  ( -1.431606283892620235, -3.149340926099361671, -3.507514324621463953 ) ) ;
#7371=CARTESIAN_POINT ( 'NONE',  ( -2.841254879263473310, -2.750659073900638685, -2.815599370228907716 ) ) ;
#7381=CARTESIAN_POINT ( 'NONE',  ( 3.007514324621436863, -0.4506590739006394175, 1.224499502706140719 ) ) ;
#7383=EDGE_CURVE ( 'NONE', #3793, #2600, #5477, .T. ) ;
#7388=CARTESIAN_POINT ( 'NONE',  ( 2.487701488670255756, -1.249340926099361093, -2.462045979635577364 ) ) ;
#7394=CARTESIAN_POINT ( 'NONE',  ( 1.638713065079161924, -3.949340926099361493, 4.007514324621467949 ) ) ;
#7398=CARTESIAN_POINT ( 'NONE',  ( 0.01814118441313990887, -1.750659073900638907, 3.500000000000000000 ) ) ;
#7402=CARTESIAN_POINT ( 'NONE',  ( 2.487701488670203354, -0.3506590739006389956, 2.462045979635629323 ) ) ;
#7408=CARTESIAN_POINT ( 'NONE',  ( -3.492485675378536047, -4.949340926099361049, -1.467888652719048670 ) ) ;
#7421=CARTESIAN_POINT ( 'NONE',  ( 0.01814118441321938349, -1.449340926099360827, -4.000000000000000000 ) ) ;
#7423=( NAMED_UNIT ( * ) PLANE_ANGLE_UNIT ( ) SI_UNIT ( $, .RADIAN. ) );
#7433=CARTESIAN_POINT ( 'NONE',  ( 3.007514324621436863, -2.050659073900639839, 1.224499502706140719 ) ) ;
#7438=CARTESIAN_POINT ( 'NONE',  ( -3.507514324621464397, -0.3493409260993610710, 1.431606283892619569 ) ) ;
#7444=CARTESIAN_POINT ( 'NONE',  ( 3.992485675378533383, -2.549340926099360694, 1.674995433905599462 ) ) ;
#7448=CARTESIAN_POINT ( 'NONE',  ( 2.487701488670203354, -6.750659073900639129, 2.462045979635629323 ) ) ;
#7452=CARTESIAN_POINT ( 'NONE',  ( -2.462045979635629323, -3.150659073900639040, 2.487701488670203798 ) ) ;
#7458=CARTESIAN_POINT ( 'NONE',  ( 3.000000000000000444, -1.049340926099361582, 0.01814118441320859698 ) ) ;
#7478=CARTESIAN_POINT ( 'NONE',  ( -1.467888652718973619, -1.050659073900638951, -3.492485675378565801 ) ) ;
#7489=SHAPE_DEFINITION_REPRESENTATION ( #8825, #1697 ) ;
#7491=CARTESIAN_POINT ( 'NONE',  ( 2.108492589042307408, -0.8493409260993616261, 2.134148098076978251 ) ) ;
#7495=CARTESIAN_POINT ( 'NONE',  ( -3.492485675378566246, -6.250659073900641793, 1.467888652718973397 ) ) ;
#7499=CARTESIAN_POINT ( 'NONE',  ( 0.01814118441313990887, -1.750659073900638907, 3.500000000000000000 ) ) ;
#7504=CARTESIAN_POINT ( 'NONE',  ( -1.224499502706077880, -3.149340926099362115, -3.007514324621463064 ) ) ;
#7516=CARTESIAN_POINT ( 'NONE',  ( 2.815599370228847320, -7.249340926099360871, 2.841254879263533262 ) ) ;
#7523=CARTESIAN_POINT ( 'NONE',  ( 1.467888652718972731, -0.2506590739006389068, 3.492485675378566246 ) ) ;
#7533=CARTESIAN_POINT ( 'NONE',  ( 3.007514324621463508, -1.149340926099361448, -1.224499502706076770 ) ) ;
#7538=CARTESIAN_POINT ( 'NONE',  ( 2.462045979635629767, -2.350659073900639218, -2.487701488670203354 ) ) ;
#7549=CARTESIAN_POINT ( 'NONE',  ( 3.007514324621463508, -4.349340926099361404, -1.224499502706076770 ) ) ;
#7554=CARTESIAN_POINT ( 'NONE',  ( -2.752888856892141689, -2.800711225422160581E-13, 1.838534025203911515 ) ) ;
#7564=CARTESIAN_POINT ( 'NONE',  ( 1.431606283892619125, -0.7493409260993610932, 3.507514324621464397 ) ) ;
#7573=CARTESIAN_POINT ( 'NONE',  ( -2.462045979635629323, -3.150659073900639040, 2.487701488670203798 ) ) ;
#7586=CARTESIAN_POINT ( 'NONE',  ( -3.507514324621464397, -6.749340926099361759, 1.431606283892619347 ) ) ;
#7589=CARTESIAN_POINT ( 'NONE',  ( -3.500000000000000000, -4.550659073900638951, 0.01814118441314012051 ) ) ;
#7594=CARTESIAN_POINT ( 'NONE',  ( -3.500000000000000000, -4.550659073900638951, 0.01814118441314012051 ) ) ;
#7600=CARTESIAN_POINT ( 'NONE',  ( 2.108492589042307408, -4.049340926099361582, 2.134148098076978251 ) ) ;
#7613=CARTESIAN_POINT ( 'NONE',  ( -1.431606283892620235, -3.149340926099361671, -3.507514324621463953 ) ) ;
#7614=CARTESIAN_POINT ( 'NONE',  ( 1.674995433905601239, -6.149340926099362115, -3.992485675378532939 ) ) ;
#7621=CARTESIAN_POINT ( 'NONE',  ( -0.01814118441314477650, -7.350659073900640550, -3.000000000000000444 ) ) ;
#7624=CARTESIAN_POINT ( 'NONE',  ( -3.500000000000000000, -8.249340926099360871, -0.01814118441321344033 ) ) ;
#7630=CARTESIAN_POINT ( 'NONE',  ( -2.462045979635576920, -4.849340926099361404, -2.487701488670255756 ) ) ;
#7634=CARTESIAN_POINT ( 'NONE',  ( 2.841254879263473310, -3.550659073900638063, 2.815599370228907272 ) ) ;
#7642=CARTESIAN_POINT ( 'NONE',  ( -0.01814118441320841310, -3.849340926099361404, 3.000000000000000444 ) ) ;
#7658=CARTESIAN_POINT ( 'NONE',  ( -3.492485675378536047, -1.749340926099361093, -1.467888652719048670 ) ) ;
#7659=CARTESIAN_POINT ( 'NONE',  ( -1.638713065079163034, -7.949340926099362825, -4.007514324621466173 ) ) ;
#7666=CARTESIAN_POINT ( 'NONE',  ( -2.992485675378564469, -6.250659073900639129, 1.260781871532430820 ) ) ;
#7676=CARTESIAN_POINT ( 'NONE',  ( -2.462045979635576920, -3.249340926099361315, -2.487701488670255756 ) ) ;
#7679=CARTESIAN_POINT ( 'NONE',  ( -4.007514324621431534, -6.050659073900639839, -1.638713065079248521 ) ) ;
#7685=CARTESIAN_POINT ( 'NONE',  ( 3.007514324621436863, -0.4506590739006394175, 1.224499502706140719 ) ) ;
#7688=MECHANICAL_DESIGN_GEOMETRIC_PRESENTATION_REPRESENTATION('',(#3826),#2798);
#7697=CARTESIAN_POINT ( 'NONE',  ( -0.01814118441321365544, -2.249340926099361315, 3.500000000000000000 ) ) ;
#7698=CARTESIAN_POINT ( 'NONE',  ( -1.467888652719046449, -0.5493409260993611376, 3.492485675378536047 ) ) ;
#7707=CARTESIAN_POINT ( 'NONE',  ( 1.674995433905515085, -1.850659073900638774, 3.992485675378568022 ) ) ;
#7718=CARTESIAN_POINT ( 'NONE',  ( -0.01814118441320841310, -3.849340926099361404, 3.000000000000000444 ) ) ;
#7721=CARTESIAN_POINT ( 'NONE',  ( -4.007514324621431534, -1.250659073900638685, -1.638713065079248521 ) ) ;
#7733=CARTESIAN_POINT ( 'NONE',  ( -3.007514324621435531, -2.850659073900640106, -1.224499502706142273 ) ) ;
#7745=CARTESIAN_POINT ( 'NONE',  ( 3.500000000000000000, -2.649340926099361226, 0.01814118441321387054 ) ) ;
#7746=CARTESIAN_POINT ( 'NONE',  ( 3.492485675378536047, -4.149340926099361226, 1.467888652719046672 ) ) ;
#7754=CARTESIAN_POINT ( 'NONE',  ( -2.815599370228907272, -1.550659073900638507, 2.841254879263473754 ) ) ;
#7758=CARTESIAN_POINT ( 'NONE',  ( -3.500000000000000000, -8.249340926099360871, -0.01814118441321344033 ) ) ;
#7763=CARTESIAN_POINT ( 'NONE',  ( 3.000000000000000444, -7.449340926099361937, 0.01814118441320859698 ) ) ;
#7767=CARTESIAN_POINT ( 'NONE',  ( -2.815599370228907272, 0.04934092609936149149, 2.841254879263473754 ) ) ;
#7778=CARTESIAN_POINT ( 'NONE',  ( 1.224499502706142273, -0.8506590739006396618, -3.007514324621435531 ) ) ;
#7786=SHAPE_REPRESENTATION_RELATIONSHIP ( 'NONE' , 'NONE' ,  #1697, #542 ) ;
#7795=CARTESIAN_POINT ( 'NONE',  ( 2.462045979635577364, -7.249340926099360871, 2.487701488670255312 ) ) ;
#7796=CARTESIAN_POINT ( 'NONE',  ( -1.431606283892620235, -6.349340926099360516, -3.507514324621463953 ) ) ;
#7802=CARTESIAN_POINT ( 'NONE',  ( 4.007514324621432422, -2.050659073900638507, 1.638713065079246078 ) ) ;
#7809=FACE_OUTER_BOUND ( 'NONE', #1858, .T. ) ;
#7811=CARTESIAN_POINT ( 'NONE',  ( 2.992485675378538712, -2.549340926099361582, 1.260781871532494103 ) ) ;
#7814=CARTESIAN_POINT ( 'NONE',  ( -3.992485675378568022, 0.1493409260993615040, 1.674995433905515529 ) ) ;
#7822=CARTESIAN_POINT ( 'NONE',  ( 3.000000000000000444, -7.449340926099361937, 0.01814118441320859698 ) ) ;
#7831=CARTESIAN_POINT ( 'NONE',  ( -3.551368067147179008, -3.053917841153461118E-13, 1.202414619655959971 ) ) ;
#7835=CARTESIAN_POINT ( 'NONE',  ( 1.467888652719048226, -6.149340926099360338, -3.492485675378536047 ) ) ;
#7843=CARTESIAN_POINT ( 'NONE',  ( 3.500000000000000000, -6.950659073900639306, -0.01814118441313969030 ) ) ;
#7851=CARTESIAN_POINT ( 'NONE',  ( 2.487701488670255756, -2.849340926099361404, -2.462045979635577364 ) ) ;
#7853=CARTESIAN_POINT ( 'NONE',  ( 2.992485675378538712, -4.149340926099362115, 1.260781871532494103 ) ) ;
#7857=CARTESIAN_POINT ( 'NONE',  ( 3.992485675378533383, -2.549340926099360694, 1.674995433905599462 ) ) ;
#7865=CARTESIAN_POINT ( 'NONE',  ( 2.992485675378565357, -2.250659073900640461, -1.260781871532430376 ) ) ;
#7870=AXIS2_PLACEMENT_3D ( 'NONE', #8889, #6051, #3186 ) ;
#7879=CARTESIAN_POINT ( 'NONE',  ( 3.500000000000000000, -7.449340926099361937, 0.01814118441321387054 ) ) ;
#7880=CARTESIAN_POINT ( 'NONE',  ( 2.487701488670255756, -6.049340926099361582, -2.462045979635577364 ) ) ;
#7881=ORIENTED_EDGE ( 'NONE', *, *, #872, .F. ) ;
#7882=FACE_OUTER_BOUND ( 'NONE', #2183, .T. ) ;
#7891=CARTESIAN_POINT ( 'NONE',  ( 2.815599370228907716, -0.7506590739006385737, -2.841254879263473310 ) ) ;
#7899=CARTESIAN_POINT ( 'NONE',  ( -2.487701488670255312, -0.4493409260993610488, 2.462045979635577808 ) ) ;
#7901=CARTESIAN_POINT ( 'NONE',  ( -2.108492589042306964, -3.249340926099361759, -2.134148098076978251 ) ) ;
#7904=CARTESIAN_POINT ( 'NONE',  ( 4.007514324621469726, -4.349340926099361404, -1.638713065079161257 ) ) ;
#7912=CARTESIAN_POINT ( 'NONE',  ( 2.134148098076933397, -3.550659073900639395, 2.108492589042352261 ) ) ;
#7920=CARTESIAN_POINT ( 'NONE',  ( 2.462045979635577364, -4.049340926099360694, 2.487701488670255312 ) ) ;
#7937=CARTESIAN_POINT ( 'NONE',  ( -0.01814118441313417734, -5.750659073900639129, -4.000000000000000000 ) ) ;
#7944=CARTESIAN_POINT ( 'NONE',  ( 3.507514324621465285, -2.749340926099361315, -1.431606283892619125 ) ) ;
#7946=CARTESIAN_POINT ( 'NONE',  ( -3.000000000000000444, -8.249340926099360871, -0.01814118441320822922 ) ) ;
#7948=CARTESIAN_POINT ( 'NONE',  ( -4.007514324621467949, -3.549340926099360694, 1.638713065079161924 ) ) ;
#7958=CARTESIAN_POINT ( 'NONE',  ( 3.000000000000000444, -6.950659073900640195, -0.01814118441314496039 ) ) ;
#7964=CARTESIAN_POINT ( 'NONE',  ( -2.462045979635576920, -6.449340926099361937, -2.487701488670255756 ) ) ;
#7976=CARTESIAN_POINT ( 'NONE',  ( -4.007514324621431534, -6.050659073900639839, -1.638713065079248521 ) ) ;
#7985=CARTESIAN_POINT ( 'NONE',  ( -2.992485675378564469, -4.650659073900640372, 1.260781871532430820 ) ) ;
#7987=CARTESIAN_POINT ( 'NONE',  ( 2.841254879263533262, -2.849340926099360960, -2.815599370228847320 ) ) ;
#7990=CARTESIAN_POINT ( 'NONE',  ( -3.500000000000000000, 0.000000000000000000, -3.665958595716611867E-14 ) ) ;
#7991=CARTESIAN_POINT ( 'NONE',  ( 3.500000000000000000, -1.049340926099360916, 0.01814118441321387054 ) ) ;
#7998=CARTESIAN_POINT ( 'NONE',  ( -3.992485675378532939, -1.749340926099360871, -1.674995433905601683 ) ) ;
#8001=CARTESIAN_POINT ( 'NONE',  ( 1.224499502706142273, -7.250659073900640905, -3.007514324621435531 ) ) ;
#8009=CARTESIAN_POINT ( 'NONE',  ( 2.487701488670255756, -6.049340926099361582, -2.462045979635577364 ) ) ;
#8022=CARTESIAN_POINT ( 'NONE',  ( -1.674995433905516196, -4.250659073900640017, -3.992485675378566690 ) ) ;
#8033=CARTESIAN_POINT ( 'NONE',  ( -2.134148098076932953, -4.350659073900638774, -2.108492589042352705 ) ) ;
#8034=UNCERTAINTY_MEASURE_WITH_UNIT (LENGTH_MEASURE( 1.000000000000000082E-05 ), #8657, 'distance_accuracy_value', 'NONE');
#8036=CARTESIAN_POINT ( 'NONE',  ( -2.815599370228846876, -3.249340926099360871, -2.841254879263533262 ) ) ;
#8040=CARTESIAN_POINT ( 'NONE',  ( 3.500000000000000000, -4.249340926099360871, 0.01814118441321387054 ) ) ;
#8045=CARTESIAN_POINT ( 'NONE',  ( -4.007514324621467949, -3.549340926099360694, 1.638713065079161924 ) ) ;
#8049=CARTESIAN_POINT ( 'NONE',  ( 1.431606283892694842, -0.8506590739006389956, -3.507514324621434199 ) ) ;
#8058=CARTESIAN_POINT ( 'NONE',  ( 3.507514324621465285, -2.749340926099361315, -1.431606283892619125 ) ) ;
#8071=CARTESIAN_POINT ( 'NONE',  ( -3.992485675378568022, -6.250659073900639129, 1.674995433905515529 ) ) ;
#8084=CARTESIAN_POINT ( 'NONE',  ( -2.992485675378564469, -1.450659073900639751, 1.260781871532430820 ) ) ;
#8088=CARTESIAN_POINT ( 'NONE',  ( -3.500000000000000000, -1.849340926099361182, -0.01814118441321344033 ) ) ;
#8094=CARTESIAN_POINT ( 'NONE',  ( 3.992485675378533383, -4.149340926099362115, 1.674995433905599462 ) ) ;
#8098=CARTESIAN_POINT ( 'NONE',  ( -3.507514324621434199, -1.250659073900638907, -1.431606283892695064 ) ) ;
#8102=CARTESIAN_POINT ( 'NONE',  ( 1.431606283892694620, -0.8506590739006389956, -3.507514324621433754 ) ) ;
#8107=CARTESIAN_POINT ( 'NONE',  ( 0.01814118441321408565, -4.649340926099361226, -3.500000000000000000 ) ) ;
#8119=CARTESIAN_POINT ( 'NONE',  ( -1.674995433905516196, -7.450659073900640195, -3.992485675378566690 ) ) ;
#8131=CARTESIAN_POINT ( 'NONE',  ( 3.000000000000000444, -0.5506590739006393953, -0.01814118441314496039 ) ) ;
#8136=CARTESIAN_POINT ( 'NONE',  ( -3.500000000000000000, 0.000000000000000000, -3.665958595716611867E-14 ) ) ;
#8137=CARTESIAN_POINT ( 'NONE',  ( -2.487701488670255312, -5.249340926099360871, 2.462045979635577808 ) ) ;
#8143=CARTESIAN_POINT ( 'NONE',  ( 4.000000000000000000, -2.649340926099360782, 0.01814118441321914063 ) ) ;
#8147=CARTESIAN_POINT ( 'NONE',  ( -3.500000000000000000, -6.150659073900639484, 0.01814118441314012051 ) ) ;
#8150=CARTESIAN_POINT ( 'NONE',  ( 3.507514324621434199, -2.050659073900638951, 1.431606283892693066 ) ) ;
#8157=CARTESIAN_POINT ( 'NONE',  ( -2.134148098076978251, -5.249340926099361759, 2.108492589042307408 ) ) ;
#8180=CARTESIAN_POINT ( 'NONE',  ( -3.500000000000000000, -1.350659073900638996, 0.01814118441314012051 ) ) ;
#8189=CARTESIAN_POINT ( 'NONE',  ( 4.007514324621469726, -5.949340926099362825, -1.638713065079161257 ) ) ;
#8192=CARTESIAN_POINT ( 'NONE',  ( -1.467888652718973619, -4.250659073900639129, -3.492485675378565801 ) ) ;
#8197=CARTESIAN_POINT ( 'NONE',  ( 2.487701488670203354, -1.950659073900639084, 2.462045979635629323 ) ) ;
#8203=CARTESIAN_POINT ( 'NONE',  ( -3.007514324621463508, -0.3493409260993614596, 1.224499502706077658 ) ) ;
#8218=CARTESIAN_POINT ( 'NONE',  ( 2.487701488670255756, -2.849340926099361404, -2.462045979635577364 ) ) ;
#8228=CARTESIAN_POINT ( 'NONE',  ( -2.462045979635629323, -1.550659073900639173, 2.487701488670203798 ) ) ;
#8237=CARTESIAN_POINT ( 'NONE',  ( 3.492485675378536047, -5.749340926099363536, 1.467888652719046672 ) ) ;
#8241=CARTESIAN_POINT ( 'NONE',  ( -3.500000000000000000, -7.750659073900639129, 0.01814118441314012051 ) ) ;
#8245=CARTESIAN_POINT ( 'NONE',  ( -1.467888652718973841, -4.250659073900638241, -3.492485675378565801 ) ) ;
#8252=CARTESIAN_POINT ( 'NONE',  ( 0.01814118441320878086, -3.049340926099361138, -3.000000000000000444 ) ) ;
#8265=CARTESIAN_POINT ( 'NONE',  ( 1.467888652719048226, -1.349340926099361182, -3.492485675378536047 ) ) ;
#8272=CARTESIAN_POINT ( 'NONE',  ( -3.492485675378566246, -3.050659073900638507, 1.467888652718973397 ) ) ;
#8276=CARTESIAN_POINT ( 'NONE',  ( 1.431606283892619347, -7.149340926099362115, 3.507514324621464397 ) ) ;
#8281=CARTESIAN_POINT ( 'NONE',  ( 1.431606283892619125, -3.949340926099361049, 3.507514324621464397 ) ) ;
#8284=CARTESIAN_POINT ( 'NONE',  ( -1.431606283892693066, -3.250659073900639129, 3.507514324621434199 ) ) ;
#8289=CARTESIAN_POINT ( 'NONE',  ( 1.467888652718972731, -3.450659073900639306, 3.492485675378566246 ) ) ;
#8295=CARTESIAN_POINT ( 'NONE',  ( -3.007514324621463508, -3.549340926099361582, 1.224499502706077658 ) ) ;
#8309=CARTESIAN_POINT ( 'NONE',  ( 3.507514324621465285, -2.749340926099361315, -1.431606283892619125 ) ) ;
#8310=CARTESIAN_POINT ( 'NONE',  ( 3.507514324621465285, -2.749340926099361315, -1.431606283892619125 ) ) ;
#8319=CARTESIAN_POINT ( 'NONE',  ( 2.487701488670203354, -1.950659073900639084, 2.462045979635629323 ) ) ;
#8330=CARTESIAN_POINT ( 'NONE',  ( -3.492485675378536047, -8.149340926099361226, -1.467888652719048670 ) ) ;
#8334=CARTESIAN_POINT ( 'NONE',  ( 3.500000000000000000, -3.750659073900639129, -0.01814118441313969030 ) ) ;
#8345=CARTESIAN_POINT ( 'NONE',  ( 0.01814118441320878086, -1.449340926099361493, -3.000000000000000444 ) ) ;
#8357=CARTESIAN_POINT ( 'NONE',  ( 2.462045979635577364, -2.449340926099361049, 2.487701488670255312 ) ) ;
#8358=CARTESIAN_POINT ( 'NONE',  ( -3.992485675378532939, -4.949340926099361937, -1.674995433905601683 ) ) ;
#8365=EDGE_CURVE ( 'NONE', #7146, #845, #4608, .T. ) ;
#8368=CARTESIAN_POINT ( 'NONE',  ( 3.507514324621434199, -3.650659073900639928, 1.431606283892693066 ) ) ;
#8377=CARTESIAN_POINT ( 'NONE',  ( 3.507514324621465285, -7.549340926099362470, -1.431606283892619125 ) ) ;
#8379=CARTESIAN_POINT ( 'NONE',  ( -1.674995433905516196, -5.850659073900638774, -3.992485675378566690 ) ) ;
#8388=CARTESIAN_POINT ( 'NONE',  ( -2.134148098076932953, -1.150659073900639040, -2.108492589042352705 ) ) ;
#8400=CARTESIAN_POINT ( 'NONE',  ( -0.01814118441321365544, -3.849340926099361404, 3.500000000000000000 ) ) ;
#8401=CARTESIAN_POINT ( 'NONE',  ( -3.992485675378532939, -8.149340926099366555, -1.674995433905601683 ) ) ;
#8409=CARTESIAN_POINT ( 'NONE',  ( -1.431606283892693066, -6.450659073900639306, 3.507514324621434199 ) ) ;
#8414=CARTESIAN_POINT ( 'NONE',  ( -2.462045979635576920, -8.049340926099361582, -2.487701488670255756 ) ) ;
#8418=CARTESIAN_POINT ( 'NONE',  ( 2.487701488670255756, -6.049340926099361582, -2.462045979635577364 ) ) ;
#8421=CARTESIAN_POINT ( 'NONE',  ( -4.000000000000000000, 0.2493409260993615095, 0.01814118441313491634 ) ) ;
#8423=CARTESIAN_POINT ( 'NONE',  ( -3.117734906886650226, -2.800711225422160581E-13, 1.098956357287211194 ) ) ;
#8429=CARTESIAN_POINT ( 'NONE',  ( -2.134148098076932953, -2.750659073900639573, -2.108492589042352705 ) ) ;
#8441=CARTESIAN_POINT ( 'NONE',  ( -3.992485675378532939, -8.149340926099366555, -1.674995433905601683 ) ) ;
#8442=CARTESIAN_POINT ( 'NONE',  ( -3.507514324621464397, -6.749340926099361759, 1.431606283892619347 ) ) ;
#8450=CARTESIAN_POINT ( 'NONE',  ( -4.000000000000000000, -1.350659073900638552, 0.01814118441313491634 ) ) ;
#8451=MANIFOLD_SOLID_BREP ( 'Cavity1', #1042 ) ;
#8463=CARTESIAN_POINT ( 'NONE',  ( 0.01814118441320878086, -4.649340926099361226, -3.000000000000000444 ) ) ;
#8466=CARTESIAN_POINT ( 'NONE',  ( 4.000000000000000000, -3.750659073900638685, -0.01814118441313441674 ) ) ;
#8477=CARTESIAN_POINT ( 'NONE',  ( 3.000000000000000444, -0.5506590739006393953, -0.01814118441314496039 ) ) ;
#8483=SURFACE_STYLE_FILL_AREA ( #2242 ) ;
#8488=CARTESIAN_POINT ( 'NONE',  ( -1.961808177976645418, 2.864554167741708363E-18, 2.934376452065968532 ) ) ;
#8490=CARTESIAN_POINT ( 'NONE',  ( 3.492485675378536047, -5.749340926099363536, 1.467888652719046672 ) ) ;
#8496=ORIENTED_EDGE ( 'NONE', *, *, #8501, .T. ) ;
#8498=CARTESIAN_POINT ( 'NONE',  ( 4.000000000000000000, -0.5506590739006383961, -0.01814118441313441674 ) ) ;
#8501=EDGE_CURVE ( 'NONE', #183, #8537, #8851, .T. ) ;
#8508=CARTESIAN_POINT ( 'NONE',  ( 3.000000000000000444, -2.649340926099361671, 0.01814118441320859698 ) ) ;
#8511=CARTESIAN_POINT ( 'NONE',  ( -1.638713065079245634, -0.05065907390063852794, 4.007514324621432422 ) ) ;
#8520=CARTESIAN_POINT ( 'NONE',  ( -1.224499502706140497, -0.05065907390063940224, 3.007514324621436863 ) ) ;
#8528=CARTESIAN_POINT ( 'NONE',  ( -2.927826432601521311, -2.017599804162953374E-16, 2.262476218830554053 ) ) ;
#8530=CARTESIAN_POINT ( 'NONE',  ( -3.500000000000000000, -8.249340926099360871, -0.01814118441321344033 ) ) ;
#8531=CARTESIAN_POINT ( 'NONE',  ( 3.500000000000000000, -7.449340926099361937, 0.01814118441321387054 ) ) ;
#8537=VERTEX_POINT ( 'NONE', #4430 ) ;
#8539=CARTESIAN_POINT ( 'NONE',  ( 3.507514324621434199, -5.250659073900640905, 1.431606283892693066 ) ) ;
#8546=CARTESIAN_POINT ( 'NONE',  ( -1.467888652719046449, -2.149340926099360782, 3.492485675378536047 ) ) ;
#8548=CARTESIAN_POINT ( 'NONE',  ( 3.000000000000000444, -4.249340926099360871, 0.01814118441320859698 ) ) ;
#8551=CARTESIAN_POINT ( 'NONE',  ( -3.992485675378568022, -4.650659073900640372, 1.674995433905515529 ) ) ;
#8559=CARTESIAN_POINT ( 'NONE',  ( -3.000000000000000444, -1.350659073900639440, 0.01814118441314532468 ) ) ;
#8565=FILL_AREA_STYLE_COLOUR ( '', #8865 ) ;
#8582=CARTESIAN_POINT ( 'NONE',  ( -0.01814118441313417734, -0.9506590739006385293, -4.000000000000000000 ) ) ;
#8590=CARTESIAN_POINT ( 'NONE',  ( -0.01814118441320841310, -2.249340926099360871, 3.000000000000000444 ) ) ;
#8594=CARTESIAN_POINT ( 'NONE',  ( -4.000000000000000000, -6.150659073900637708, 0.01814118441313491634 ) ) ;
#8603=CARTESIAN_POINT ( 'NONE',  ( 1.224499502706142273, -4.050659073900639839, -3.007514324621435531 ) ) ;
#8613=CARTESIAN_POINT ( 'NONE',  ( 3.492485675378536047, -5.749340926099363536, 1.467888652719046672 ) ) ;
#8617=CARTESIAN_POINT ( 'NONE',  ( 3.500000000000000000, -4.249340926099360871, 0.01814118441321387054 ) ) ;
#8619=CARTESIAN_POINT ( 'NONE',  ( -3.500000000000000000, -7.750659073900639129, 0.01814118441314011704 ) ) ;
#8627=CARTESIAN_POINT ( 'NONE',  ( -4.007514324621467949, -0.3493409260993607379, 1.638713065079161924 ) ) ;
#8636=CARTESIAN_POINT ( 'NONE',  ( 3.492485675378536047, -2.549340926099360694, 1.467888652719046672 ) ) ;
#8637=CARTESIAN_POINT ( 'NONE',  ( -0.01814118441314477650, -0.9506590739006395285, -3.000000000000000444 ) ) ;
#8639=CARTESIAN_POINT ( 'NONE',  ( 3.992485675378568910, -7.050659073900638063, -1.674995433905514863 ) ) ;
#8651=CARTESIAN_POINT ( 'NONE',  ( 3.007514324621436863, -5.250659073900640017, 1.224499502706140719 ) ) ;
#8657=( LENGTH_UNIT ( ) NAMED_UNIT ( * ) SI_UNIT ( .MILLI., .METRE. ) );
#8660=CARTESIAN_POINT ( 'NONE',  ( 1.467888652719048226, -6.149340926099360338, -3.492485675378536047 ) ) ;
#8675=CARTESIAN_POINT ( 'NONE',  ( -1.638713065079245634, -4.850659073900639662, 4.007514324621432422 ) ) ;
#8678=CARTESIAN_POINT ( 'NONE',  ( -3.500000000000000000, -7.750659073900639129, 0.01814118441314011704 ) ) ;
#8682=CARTESIAN_POINT ( 'NONE',  ( 0.01814118441321408565, -1.449340926099361271, -3.500000000000000000 ) ) ;
#8684=CARTESIAN_POINT ( 'NONE',  ( -2.992485675378564469, -3.050659073900639839, 1.260781871532430820 ) ) ;
#8687=CARTESIAN_POINT ( 'NONE',  ( 1.674995433905601239, -2.949340926099360605, -3.992485675378532939 ) ) ;
#8690=CARTESIAN_POINT ( 'NONE',  ( -3.492485675378535603, -3.349340926099361404, -1.467888652719048670 ) ) ;
#8695=CARTESIAN_POINT ( 'NONE',  ( -1.674995433905599462, -6.949340926099362825, 3.992485675378533383 ) ) ;
#8699=CARTESIAN_POINT ( 'NONE',  ( -3.500000000000000000, 0.2493409260993610654, 0.01814118441314012051 ) ) ;
#8706=CARTESIAN_POINT ( 'NONE',  ( -0.01814118441321365544, -3.849340926099361404, 3.500000000000000000 ) ) ;
#8709=CARTESIAN_POINT ( 'NONE',  ( 2.487701488670255756, -7.649340926099361226, -2.462045979635577364 ) ) ;
#8718=CARTESIAN_POINT ( 'NONE',  ( -1.638713065079245634, -3.250659073900639129, 4.007514324621432422 ) ) ;
#8730=CARTESIAN_POINT ( 'NONE',  ( 2.992485675378565357, -3.850659073900639662, -1.260781871532430376 ) ) ;
#8733=CARTESIAN_POINT ( 'NONE',  ( 1.638713065079161924, -2.349340926099360960, 4.007514324621467949 ) ) ;
#8736=CARTESIAN_POINT ( 'NONE',  ( -2.462045979635576920, -4.849340926099361404, -2.487701488670255756 ) ) ;
#8740=CARTESIAN_POINT ( 'NONE',  ( 1.638713065079161924, -2.349340926099360960, 4.007514324621467949 ) ) ;
#8744=CARTESIAN_POINT ( 'NONE',  ( -2.108492589042352261, -4.750659073900640017, 2.134148098076933397 ) ) ;
#8751=ADVANCED_FACE ( 'NONE', ( #6007 ), #8846, .F. ) ;
#8755=CARTESIAN_POINT ( 'NONE',  ( 1.467888652719048226, -4.549340926099360694, -3.492485675378536047 ) ) ;
#8767=CARTESIAN_POINT ( 'NONE',  ( -0.01814118441313417734, -2.550659073900638951, -4.000000000000000000 ) ) ;
#8778=CARTESIAN_POINT ( 'NONE',  ( -2.108492589042352261, -1.550659073900639395, 2.134148098076933397 ) ) ;
#8784=CARTESIAN_POINT ( 'NONE',  ( -3.492485675378535603, -1.749340926099361093, -1.467888652719048670 ) ) ;
#8788=CARTESIAN_POINT ( 'NONE',  ( 4.000000000000000000, -7.449340926099361937, 0.01814118441321914063 ) ) ;
#8792=CARTESIAN_POINT ( 'NONE',  ( -1.260781871532431708, -7.450659073900640195, -2.992485675378564469 ) ) ;
#8795=CARTESIAN_POINT ( 'NONE',  ( -2.487701488670202910, -4.350659073900638774, -2.462045979635629767 ) ) ;
#8800=CARTESIAN_POINT ( 'NONE',  ( -3.507514324621464397, -1.949340926099361271, 1.431606283892619347 ) ) ;
#8812=CARTESIAN_POINT ( 'NONE',  ( -1.638713065079245634, -6.450659073900638418, 4.007514324621432422 ) ) ;
#8823=CARTESIAN_POINT ( 'NONE',  ( 2.134148098076933397, -0.3506590739006394397, 2.108492589042352261 ) ) ;
#8825=PRODUCT_DEFINITION_SHAPE ( 'NONE', 'NONE',  #5115 ) ;
#8828=CARTESIAN_POINT ( 'NONE',  ( -1.431606283892620235, -4.749340926099363536, -3.507514324621463953 ) ) ;
#8832=CARTESIAN_POINT ( 'NONE',  ( 2.841254879263533262, -7.649340926099361226, -2.815599370228847320 ) ) ;
#8836=CARTESIAN_POINT ( 'NONE',  ( 1.431606283892694842, -7.250659073900640017, -3.507514324621434199 ) ) ;
#8839=CARTESIAN_POINT ( 'NONE',  ( -3.492485675378566246, -1.450659073900639084, 1.467888652718973175 ) ) ;
#8845=CARTESIAN_POINT ( 'NONE',  ( -2.108492589042306964, -4.849340926099359628, -2.134148098076978251 ) ) ;
#8846=PLANE ( 'NONE',  #7870 ) ;
#8849=CARTESIAN_POINT ( 'NONE',  ( -1.926921503246612044, -5.459919674188128654E-16, 2.888980742429482884 ) ) ;
#8851=B_SPLINE_CURVE_WITH_KNOTS ( 'NONE', 3,
 ( #5554, #1410, #6333, #8488, #4250, #7083, #705, #3554, #59, #6375, #5681, #2863, #15, #8528, #4976, #1980, #7831, #1449, #3597, #6421 ),
 .UNSPECIFIED., .F., .F.,
 ( 4, 2, 2, 2, 2, 2, 2, 2, 2, 4 ),
 ( 0.003307978161309543027, 0.003337183750601276089, 0.003366389339893009151, 0.003424800518476474841, 0.003541622875643406221, 0.003775267589977268981, 0.004242557018644994501, 0.005177135875980443808, 0.006111714733315892246, 0.007046293590651341553 ),
 .UNSPECIFIED. ) ;
#8863=CARTESIAN_POINT ( 'NONE',  ( -3.492485675378566246, 0.1493409260993610876, 1.467888652718973397 ) ) ;
#8865=COLOUR_RGB ( '',0.8941176470588234615, 0.8941176470588234615, 0.8941176470588234615 ) ;
#8868=CARTESIAN_POINT ( 'NONE',  ( -1.467888652719046449, -5.349340926099361404, 3.492485675378535603 ) ) ;
#8873=CARTESIAN_POINT ( 'NONE',  ( -1.674995433905599462, -3.749340926099360871, 3.992485675378533383 ) ) ;
#8876=CARTESIAN_POINT ( 'NONE',  ( -3.492485675378566246, -3.050659073900638507, 1.467888652718973397 ) ) ;
#8879=CARTESIAN_POINT ( 'NONE',  ( -1.467888652718973841, -7.450659073900639306, -3.492485675378565801 ) ) ;
#8880=CARTESIAN_POINT ( 'NONE',  ( 3.507514324621434199, -3.650659073900639484, 1.431606283892693066 ) ) ;
#8888=CARTESIAN_POINT ( 'NONE',  ( 2.134148098076978251, -2.849340926099362292, -2.108492589042307408 ) ) ;
#8889=CARTESIAN_POINT ( 'NONE',  ( -3.500000000000000000, -7.750659073900639129, 0.01814118441314012051 ) ) ;
#8901=CARTESIAN_POINT ( 'NONE',  ( 4.000000000000000000, -7.449340926099361937, 0.01814118441321914063 ) ) ;
#8910=CARTESIAN_POINT ( 'NONE',  ( 3.507514324621434199, -0.4506590739006390844, 1.431606283892693066 ) ) ;
#8920=CARTESIAN_POINT ( 'NONE',  ( -3.500000000000000000, -8.249340926099360871, -0.01814118441321344033 ) ) ;
#8923=CARTESIAN_POINT ( 'NONE',  ( -1.467888652718973619, -7.450659073900638418, -3.492485675378565801 ) ) ;
#8933=CARTESIAN_POINT ( 'NONE',  ( 1.260781871532495657, -4.549340926099363358, -2.992485675378538268 ) ) ;
#8945=CARTESIAN_POINT ( 'NONE',  ( -3.500000000000000000, 0.000000000000000000, -3.665958595716611867E-14 ) ) ;
#8947=CARTESIAN_POINT ( 'NONE',  ( -2.487701488670255312, -2.049340926099361582, 2.462045979635577808 ) ) ;
#8957=CARTESIAN_POINT ( 'NONE',  ( -2.487701488670202910, -2.750659073900639129, -2.462045979635629767 ) ) ;
#8968=CARTESIAN_POINT ( 'NONE',  ( 2.462045979635577364, -7.249340926099360871, 2.487701488670255312 ) ) ;
#8971=CARTESIAN_POINT ( 'NONE',  ( -1.467888652718973619, -2.650659073900639040, -3.492485675378565801 ) ) ;
#8976=CARTESIAN_POINT ( 'NONE',  ( -2.462045979635629323, -1.550659073900639173, 2.487701488670203798 ) ) ;
#8982=CARTESIAN_POINT ( 'NONE',  ( -3.000000000000000444, -5.049340926099361582, -0.01814118441320822922 ) ) ;
#8994=CARTESIAN_POINT ( 'NONE',  ( -2.815599370228846876, -8.049340926099359805, -2.841254879263533262 ) ) ;
#8995=CARTESIAN_POINT ( 'NONE',  ( 3.492485675378536047, -2.549340926099360694, 1.467888652719046672 ) ) ;
#9004=CARTESIAN_POINT ( 'NONE',  ( 0.01814118441313990887, -1.750659073900638907, 3.500000000000000000 ) ) ;
#9015=CARTESIAN_POINT ( 'NONE',  ( 1.467888652719048226, -7.749340926099361759, -3.492485675378536047 ) ) ;
#9018=CARTESIAN_POINT ( 'NONE',  ( 1.467888652718972731, -6.650659073900639484, 3.492485675378566246 ) ) ;
#9019=ORIENTED_EDGE ( 'NONE', *, *, #3658, .T. ) ;
#9022=CARTESIAN_POINT ( 'NONE',  ( 2.462045979635629767, -5.550659073900639839, -2.487701488670203354 ) ) ;
#9027=CARTESIAN_POINT ( 'NONE',  ( 2.992485675378538712, -0.9493409260993616039, 1.260781871532494103 ) ) ;
#9042=CARTESIAN_POINT ( 'NONE',  ( 2.487701488670255756, -1.249340926099361093, -2.462045979635577364 ) ) ;
#9043=CARTESIAN_POINT ( 'NONE',  ( -3.507514324621464397, -1.949340926099361271, 1.431606283892619347 ) ) ;
#9051=CARTESIAN_POINT ( 'NONE',  ( 1.467888652718972731, -1.850659073900638996, 3.492485675378566246 ) ) ;
#9063=CARTESIAN_POINT ( 'NONE',  ( 0.01814118441321408565, -6.249340926099360871, -3.500000000000000000 ) ) ;
#9067=CARTESIAN_POINT ( 'NONE',  ( 3.992485675378568910, -0.6506590739006385959, -1.674995433905514863 ) ) ;
#9076=CARTESIAN_POINT ( 'NONE',  ( -3.000000000000000444, -8.249340926099360871, -0.01814118441320822922 ) ) ;
#9081=DIRECTION ( 'NONE',  ( 0.000000000000000000, 0.000000000000000000, 1.000000000000000000 ) ) ;
#9088=CARTESIAN_POINT ( 'NONE',  ( 0.01814118441321408565, -3.049340926099361138, -3.500000000000000000 ) ) ;
#9089=CARTESIAN_POINT ( 'NONE',  ( 1.638713065079161924, -5.549340926099361582, 4.007514324621467949 ) ) ;
#9094=ORIENTED_EDGE ( 'NONE', *, *, #7383, .F. ) ;
#9096=CARTESIAN_POINT ( 'NONE',  ( -3.492485675378566246, -6.250659073900641793, 1.467888652718973397 ) ) ;
#9107=CARTESIAN_POINT ( 'NONE',  ( -0.01814118441320841310, -0.6493409260993614485, 3.000000000000000444 ) ) ;
#9111=CARTESIAN_POINT ( 'NONE',  ( 4.007514324621432422, -3.650659073900639040, 1.638713065079246078 ) ) ;
#9120=CARTESIAN_POINT ( 'NONE',  ( -0.01814118441314477650, -2.550659073900638951, -3.000000000000000444 ) ) ;
#9132=CARTESIAN_POINT ( 'NONE',  ( 2.462045979635577364, -4.049340926099360694, 2.487701488670255312 ) ) ;
#9133=CARTESIAN_POINT ( 'NONE',  ( -3.500000000000000000, -8.249340926099360871, -0.01814118441321344033 ) ) ;
#9141=CARTESIAN_POINT ( 'NONE',  ( -1.638713065079245634, -0.05065907390063852794, 4.007514324621432422 ) ) ;
#9149=CARTESIAN_POINT ( 'NONE',  ( -0.01814118441320841310, -7.049340926099361582, 3.000000000000000444 ) ) ;
#9152=CARTESIAN_POINT ( 'NONE',  ( 4.007514324621432422, -2.050659073900638507, 1.638713065079246078 ) ) ;
#9159=CARTESIAN_POINT ( 'NONE',  ( -3.007514324621435531, -1.250659073900639573, -1.224499502706142273 ) ) ;
#9170=( NAMED_UNIT ( * ) SI_UNIT ( $, .STERADIAN. ) SOLID_ANGLE_UNIT ( ) );
#9172=CARTESIAN_POINT ( 'NONE',  ( 1.467888652719048226, -1.349340926099361182, -3.492485675378536047 ) ) ;
#9173=CARTESIAN_POINT ( 'NONE',  ( -1.431606283892620235, -7.949340926099361049, -3.507514324621463953 ) ) ;
#9179=CARTESIAN_POINT ( 'NONE',  ( -0.01814118441313947866, -7.350659073900638774, -3.500000000000000000 ) ) ;
#9219=COLOUR_RGB('Grey',0.48,0.52,0.57);
#9220=FILL_AREA_STYLE_COLOUR('',#9219);
#9221=FILL_AREA_STYLE('',(#9220));
#9222=SURFACE_STYLE_FILL_AREA(#9221);
#9223=SURFACE_SIDE_STYLE('',(#9222));
#9224=SURFACE_STYLE_USAGE(.BOTH.,#9223);
#9225=PRESENTATION_STYLE_ASSIGNMENT((#9224));
ENDSEC;
END-ISO-10303-21;
